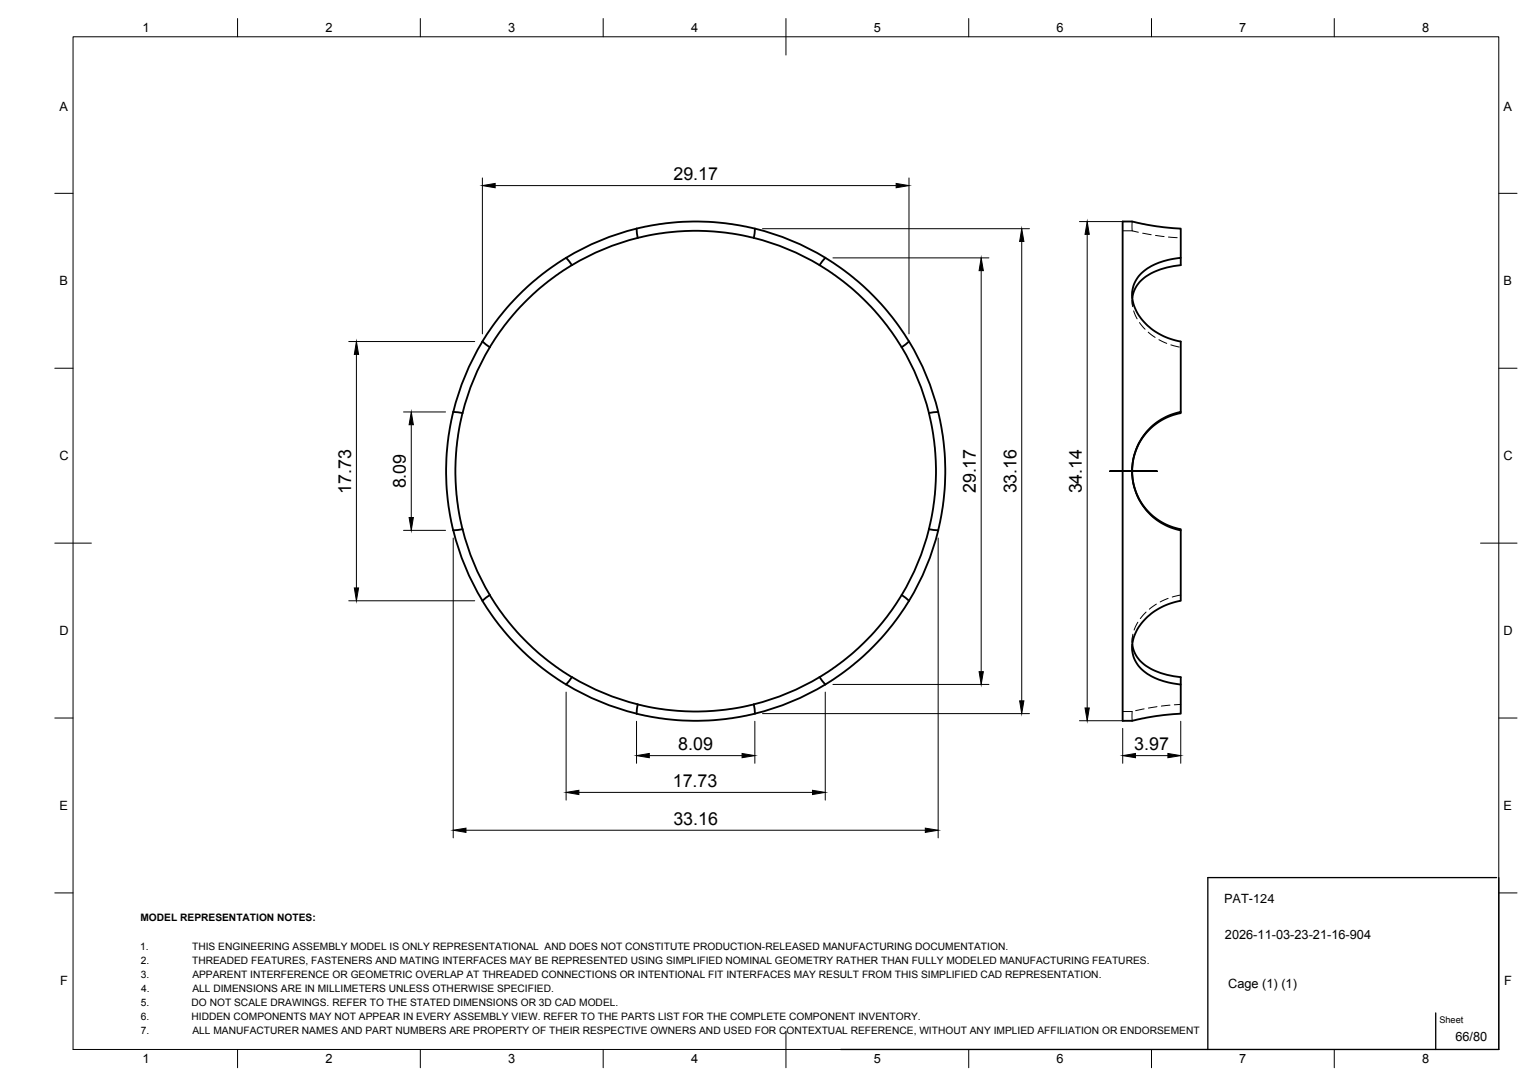
ISO-10303-21;
HEADER;
/* Generated by software containing ST-Developer
 * from STEP Tools, Inc. (www.steptools.com) 
 */

FILE_DESCRIPTION(
/* description */ ('XY cross-slide table'),
/* implementation_level */ '2;1');

FILE_NAME(
/* name */ 'Cage (1) (1).step',
/* time_stamp */ '2026-10-28T03:22:46-07:00',
/* author */ (''),
/* organization */ (''),
/* preprocessor_version */ 'ST-DEVELOPER v20.2',
/* originating_system */ 'Autodesk Translation Framework v15.17.0.0',
/* authorisation */ '');

FILE_SCHEMA (('AUTOMOTIVE_DESIGN { 1 0 10303 214 3 1 1 }'));
ENDSEC;

DATA;
#10=MECHANICAL_DESIGN_GEOMETRIC_PRESENTATION_REPRESENTATION('',(#1758),#62984);
#1051=B_SPLINE_CURVE_WITH_KNOTS('',3,(#49166,#49167,#49168,#49169,#49170,
#49171,#49172,#49173,#49174,#49175,#49176,#49177,#49178,#49179,#49180,#49181,
#49182,#49183,#49184,#49185,#49186,#49187),.UNSPECIFIED.,.F.,.F.,(4,2,2,
2,2,2,2,2,2,2,4),(0.0789094028588958,0.210573405340968,0.315860108011452,
0.421146810681936,0.522142632548711,0.623138454415485,0.72413427628226,
0.825130098149035,0.930416800819519,1.03570350349,1.16736750597208),
 .UNSPECIFIED.);
#1052=B_SPLINE_CURVE_WITH_KNOTS('',3,(#49191,#49192,#49193,#49194,#49195,
#49196,#49197,#49198,#49199,#49200,#49201,#49202,#49203,#49204,#49205,#49206,
#49207,#49208,#49209,#49210,#49211,#49212),.UNSPECIFIED.,.F.,.F.,(4,2,2,
2,2,2,2,2,2,2,4),(0.0774793363974613,0.142088896491891,0.284177792983782,
0.411119756996526,0.514392970548519,0.617666184100513,0.720939397652506,
0.8242126112045,0.951154575217244,1.09324347170913,1.15785303180356),
 .UNSPECIFIED.);
#1053=B_SPLINE_CURVE_WITH_KNOTS('',3,(#49218,#49219,#49220,#49221,#49222,
#49223,#49224,#49225,#49226,#49227,#49228,#49229,#49230,#49231,#49232,#49233,
#49234,#49235,#49236,#49237,#49238,#49239),.UNSPECIFIED.,.F.,.F.,(4,2,2,
2,2,2,2,2,2,2,4),(0.0774793363974613,0.142088896491891,0.284177792983782,
0.411119756996525,0.514392970548519,0.617666184100513,0.720939397652506,
0.8242126112045,0.951154575217243,1.09324347170913,1.15785303180356),
 .UNSPECIFIED.);
#1054=B_SPLINE_CURVE_WITH_KNOTS('',3,(#49243,#49244,#49245,#49246,#49247,
#49248,#49249,#49250,#49251,#49252,#49253,#49254,#49255,#49256,#49257,#49258,
#49259,#49260,#49261,#49262,#49263,#49264),.UNSPECIFIED.,.F.,.F.,(4,2,2,
2,2,2,2,2,2,2,4),(0.0774793363974614,0.142088896491891,0.284177792983781,
0.411119756996525,0.514392970548519,0.617666184100512,0.720939397652506,
0.824212611204499,0.951154575217243,1.09324347170913,1.15785303180356),
 .UNSPECIFIED.);
#1055=B_SPLINE_CURVE_WITH_KNOTS('',3,(#49268,#49269,#49270,#49271,#49272,
#49273,#49274,#49275,#49276,#49277,#49278,#49279),.UNSPECIFIED.,.F.,.F.,
(4,2,2,2,2,4),(0.0774793363974613,0.142088896491891,0.284177792983781,0.411119756996525,
0.514392970548519,0.617666184100512),.UNSPECIFIED.);
#1056=B_SPLINE_CURVE_WITH_KNOTS('',3,(#49284,#49285,#49286,#49287,#49288,
#49289,#49290,#49291,#49292,#49293,#49294,#49295),.UNSPECIFIED.,.F.,.F.,
(4,2,2,2,2,4),(0.617666184100512,0.720939397652506,0.824212611204499,0.951154575217243,
1.09324347170913,1.15785303180356),.UNSPECIFIED.);
#1057=B_SPLINE_CURVE_WITH_KNOTS('',3,(#49299,#49300,#49301,#49302,#49303,
#49304,#49305,#49306,#49307,#49308,#49309,#49310,#49311,#49312,#49313,#49314,
#49315,#49316,#49317,#49318,#49319,#49320),.UNSPECIFIED.,.F.,.F.,(4,2,2,
2,2,2,2,2,2,2,4),(0.0774793363974613,0.142088896491891,0.284177792983782,
0.411119756996526,0.514392970548519,0.617666184100513,0.720939397652507,
0.8242126112045,0.951154575217245,1.09324347170914,1.15785303180356),
 .UNSPECIFIED.);
#1058=B_SPLINE_CURVE_WITH_KNOTS('',3,(#49324,#49325,#49326,#49327,#49328,
#49329,#49330,#49331,#49332,#49333,#49334,#49335,#49336,#49337,#49338,#49339,
#49340,#49341,#49342,#49343,#49344,#49345),.UNSPECIFIED.,.F.,.F.,(4,2,2,
2,2,2,2,2,2,2,4),(0.0774793363974613,0.142088896491891,0.284177792983782,
0.411119756996526,0.514392970548519,0.617666184100513,0.720939397652506,
0.824212611204499,0.951154575217243,1.09324347170913,1.15785303180356),
 .UNSPECIFIED.);
#1059=B_SPLINE_CURVE_WITH_KNOTS('',3,(#49349,#49350,#49351,#49352,#49353,
#49354,#49355,#49356,#49357,#49358,#49359,#49360,#49361,#49362,#49363,#49364,
#49365,#49366,#49367,#49368,#49369,#49370),.UNSPECIFIED.,.F.,.F.,(4,2,2,
2,2,2,2,2,2,2,4),(0.0774793363974613,0.142088896491891,0.284177792983782,
0.411119756996526,0.514392970548519,0.617666184100513,0.720939397652506,
0.8242126112045,0.951154575217244,1.09324347170913,1.15785303180356),
 .UNSPECIFIED.);
#1060=B_SPLINE_CURVE_WITH_KNOTS('',3,(#49374,#49375,#49376,#49377,#49378,
#49379,#49380,#49381,#49382,#49383,#49384,#49385,#49386,#49387,#49388,#49389,
#49390,#49391,#49392,#49393,#49394,#49395),.UNSPECIFIED.,.F.,.F.,(4,2,2,
2,2,2,2,2,2,2,4),(0.0774793363974613,0.142088896491891,0.284177792983782,
0.411119756996526,0.514392970548519,0.617666184100513,0.720939397652506,
0.8242126112045,0.951154575217243,1.09324347170913,1.15785303180356),
 .UNSPECIFIED.);
#1061=B_SPLINE_CURVE_WITH_KNOTS('',3,(#49403,#49404,#49405,#49406,#49407,
#49408,#49409,#49410,#49411,#49412,#49413,#49414,#49415,#49416,#49417,#49418,
#49419,#49420,#49421,#49422,#49423,#49424),.UNSPECIFIED.,.F.,.F.,(4,2,2,
2,2,2,2,2,2,2,4),(0.0789094028588958,0.210573405340968,0.315860108011452,
0.421146810681936,0.522142632548711,0.623138454415485,0.72413427628226,
0.825130098149035,0.930416800819519,1.03570350349,1.16736750597208),
 .UNSPECIFIED.);
#1062=B_SPLINE_CURVE_WITH_KNOTS('',3,(#49432,#49433,#49434,#49435,#49436,
#49437,#49438,#49439,#49440,#49441,#49442,#49443,#49444,#49445,#49446,#49447,
#49448,#49449,#49450,#49451,#49452,#49453),.UNSPECIFIED.,.F.,.F.,(4,2,2,
2,2,2,2,2,2,2,4),(0.0789094028588958,0.210573405340969,0.315860108011453,
0.421146810681937,0.522142632548712,0.623138454415486,0.724134276282261,
0.825130098149035,0.930416800819519,1.03570350349,1.16736750597208),
 .UNSPECIFIED.);
#1063=B_SPLINE_CURVE_WITH_KNOTS('',3,(#49462,#49463,#49464,#49465,#49466,
#49467,#49468,#49469,#49470,#49471,#49472,#49473),.UNSPECIFIED.,.F.,.F.,
(4,2,2,2,2,4),(0.0789094028588958,0.210573405340968,0.315860108011452,0.421146810681937,
0.522142632548711,0.623138454415486),.UNSPECIFIED.);
#1064=B_SPLINE_CURVE_WITH_KNOTS('',3,(#49475,#49476,#49477,#49478,#49479,
#49480,#49481,#49482,#49483,#49484,#49485,#49486),.UNSPECIFIED.,.F.,.F.,
(4,2,2,2,2,4),(0.623138454415486,0.72413427628226,0.825130098149035,0.930416800819519,
1.03570350349,1.16736750597208),.UNSPECIFIED.);
#1065=B_SPLINE_CURVE_WITH_KNOTS('',3,(#49493,#49494,#49495,#49496,#49497,
#49498,#49499,#49500,#49501,#49502,#49503,#49504,#49505,#49506,#49507,#49508,
#49509,#49510,#49511,#49512,#49513,#49514),.UNSPECIFIED.,.F.,.F.,(4,2,2,
2,2,2,2,2,2,2,4),(0.0789094028588958,0.210573405340968,0.315860108011452,
0.421146810681936,0.522142632548711,0.623138454415486,0.72413427628226,
0.825130098149035,0.930416800819519,1.03570350349,1.16736750597208),
 .UNSPECIFIED.);
#1066=B_SPLINE_CURVE_WITH_KNOTS('',3,(#49522,#49523,#49524,#49525,#49526,
#49527,#49528,#49529,#49530,#49531,#49532,#49533,#49534,#49535,#49536,#49537,
#49538,#49539,#49540,#49541,#49542,#49543),.UNSPECIFIED.,.F.,.F.,(4,2,2,
2,2,2,2,2,2,2,4),(0.0789094028588957,0.210573405340968,0.315860108011452,
0.421146810681936,0.522142632548711,0.623138454415485,0.72413427628226,
0.825130098149035,0.930416800819519,1.03570350349,1.16736750597207),
 .UNSPECIFIED.);
#1067=B_SPLINE_CURVE_WITH_KNOTS('',3,(#49551,#49552,#49553,#49554,#49555,
#49556,#49557,#49558,#49559,#49560,#49561,#49562,#49563,#49564,#49565,#49566,
#49567,#49568,#49569,#49570,#49571,#49572),.UNSPECIFIED.,.F.,.F.,(4,2,2,
2,2,2,2,2,2,2,4),(0.0789094028588958,0.210573405340968,0.315860108011452,
0.421146810681936,0.522142632548711,0.623138454415486,0.72413427628226,
0.825130098149035,0.930416800819519,1.03570350349,1.16736750597208),
 .UNSPECIFIED.);
#1068=B_SPLINE_CURVE_WITH_KNOTS('',3,(#49581,#49582,#49583,#49584,#49585,
#49586,#49587,#49588,#49589,#49590,#49591,#49592,#49593,#49594,#49595,#49596,
#49597,#49598,#49599,#49600,#49601,#49602),.UNSPECIFIED.,.F.,.F.,(4,2,2,
2,2,2,2,2,2,2,4),(0.0789094028588958,0.210573405340968,0.315860108011452,
0.421146810681936,0.522142632548711,0.623138454415485,0.72413427628226,
0.825130098149035,0.930416800819519,1.03570350349,1.16736750597208),
 .UNSPECIFIED.);
#1433=SPHERICAL_SURFACE('',#25717,0.412776);
#1434=SPHERICAL_SURFACE('',#25733,0.412776);
#1435=SPHERICAL_SURFACE('',#25738,0.412776);
#1436=SPHERICAL_SURFACE('',#25743,0.412776);
#1437=SPHERICAL_SURFACE('',#25748,0.412776);
#1438=SPHERICAL_SURFACE('',#25753,0.412776);
#1439=SPHERICAL_SURFACE('',#25758,0.412776);
#1440=SPHERICAL_SURFACE('',#25766,0.412776);
#1563=SHAPE_REPRESENTATION_RELATIONSHIP('SRR','None',#63420,#1646);
#1646=ADVANCED_BREP_SHAPE_REPRESENTATION('',(#1867),#62957);
#1758=STYLED_ITEM('',(#63926),#1867);
#1867=MANIFOLD_SOLID_BREP('Continuous crown cage',#23056);
#2214=FACE_BOUND('',#5406,.T.);
#2682=PLANE('',#25730);
#2683=PLANE('',#25735);
#2684=PLANE('',#25740);
#2685=PLANE('',#25745);
#2686=PLANE('',#25750);
#2687=PLANE('',#25755);
#2688=PLANE('',#25764);
#2689=PLANE('',#25768);
#2690=PLANE('',#25769);
#3747=FACE_OUTER_BOUND('',#5388,.T.);
#3748=FACE_OUTER_BOUND('',#5389,.T.);
#3749=FACE_OUTER_BOUND('',#5390,.T.);
#3750=FACE_OUTER_BOUND('',#5391,.T.);
#3751=FACE_OUTER_BOUND('',#5392,.T.);
#3752=FACE_OUTER_BOUND('',#5393,.T.);
#3753=FACE_OUTER_BOUND('',#5394,.T.);
#3754=FACE_OUTER_BOUND('',#5395,.T.);
#3755=FACE_OUTER_BOUND('',#5396,.T.);
#3756=FACE_OUTER_BOUND('',#5397,.T.);
#3757=FACE_OUTER_BOUND('',#5398,.T.);
#3758=FACE_OUTER_BOUND('',#5399,.T.);
#3759=FACE_OUTER_BOUND('',#5400,.T.);
#3760=FACE_OUTER_BOUND('',#5401,.T.);
#3761=FACE_OUTER_BOUND('',#5402,.T.);
#3762=FACE_OUTER_BOUND('',#5403,.T.);
#3763=FACE_OUTER_BOUND('',#5404,.T.);
#3764=FACE_OUTER_BOUND('',#5405,.T.);
#3765=FACE_OUTER_BOUND('',#5407,.T.);
#5388=EDGE_LOOP('',(#18906,#18907,#18908,#18909));
#5389=EDGE_LOOP('',(#18910,#18911,#18912,#18913,#18914,#18915,#18916,#18917,
#18918,#18919,#18920,#18921,#18922,#18923,#18924,#18925,#18926,#18927,#18928,
#18929));
#5390=EDGE_LOOP('',(#18930,#18931,#18932,#18933));
#5391=EDGE_LOOP('',(#18934,#18935,#18936,#18937));
#5392=EDGE_LOOP('',(#18938,#18939,#18940,#18941));
#5393=EDGE_LOOP('',(#18942,#18943,#18944,#18945));
#5394=EDGE_LOOP('',(#18946,#18947,#18948,#18949));
#5395=EDGE_LOOP('',(#18950,#18951,#18952,#18953,#18954,#18955));
#5396=EDGE_LOOP('',(#18956,#18957,#18958,#18959));
#5397=EDGE_LOOP('',(#18960,#18961,#18962,#18963));
#5398=EDGE_LOOP('',(#18964,#18965,#18966,#18967));
#5399=EDGE_LOOP('',(#18968,#18969,#18970,#18971));
#5400=EDGE_LOOP('',(#18972,#18973,#18974,#18975));
#5401=EDGE_LOOP('',(#18976,#18977,#18978,#18979));
#5402=EDGE_LOOP('',(#18980,#18981,#18982,#18983,#18984,#18985,#18986,#18987,
#18988,#18989,#18990,#18991,#18992,#18993,#18994,#18995,#18996,#18997,#18998,
#18999));
#5403=EDGE_LOOP('',(#19000,#19001,#19002,#19003));
#5404=EDGE_LOOP('',(#19004,#19005,#19006,#19007));
#5405=EDGE_LOOP('',(#19008));
#5406=EDGE_LOOP('',(#19009));
#5407=EDGE_LOOP('',(#19010,#19011,#19012,#19013));
#6863=LINE('',#49281,#8350);
#6864=LINE('',#49577,#8351);
#8350=VECTOR('',#30866,1.706752);
#8351=VECTOR('',#30943,1.643248);
#9566=CIRCLE('',#25718,0.405071403305639);
#9567=CIRCLE('',#25719,0.405071403305639);
#9568=CIRCLE('',#25721,1.706752);
#9569=CIRCLE('',#25722,1.706752);
#9570=CIRCLE('',#25723,1.706752);
#9571=CIRCLE('',#25724,1.706752);
#9572=CIRCLE('',#25725,1.706752);
#9573=CIRCLE('',#25726,1.706752);
#9574=CIRCLE('',#25727,1.706752);
#9575=CIRCLE('',#25728,1.706752);
#9576=CIRCLE('',#25729,1.706752);
#9577=CIRCLE('',#25731,1.643248);
#9578=CIRCLE('',#25732,0.405071403305639);
#9579=CIRCLE('',#25734,0.405071403305639);
#9580=CIRCLE('',#25736,1.643248);
#9581=CIRCLE('',#25737,0.405071403305639);
#9582=CIRCLE('',#25739,0.405071403305639);
#9583=CIRCLE('',#25741,1.643248);
#9584=CIRCLE('',#25742,0.405071403305639);
#9585=CIRCLE('',#25744,0.405071403305639);
#9586=CIRCLE('',#25746,1.643248);
#9587=CIRCLE('',#25747,0.405071403305639);
#9588=CIRCLE('',#25749,0.405071403305639);
#9589=CIRCLE('',#25751,1.643248);
#9590=CIRCLE('',#25752,0.405071403305639);
#9591=CIRCLE('',#25754,0.405071403305639);
#9592=CIRCLE('',#25756,1.643248);
#9593=CIRCLE('',#25757,0.405071403305639);
#9594=CIRCLE('',#25759,0.405071403305639);
#9595=CIRCLE('',#25761,1.643248);
#9596=CIRCLE('',#25762,1.643248);
#9597=CIRCLE('',#25763,1.643248);
#9598=CIRCLE('',#25765,0.405071403305639);
#9599=CIRCLE('',#25767,0.405071403305639);
#11131=VERTEX_POINT('',#49164);
#11132=VERTEX_POINT('',#49165);
#11133=VERTEX_POINT('',#49188);
#11134=VERTEX_POINT('',#49190);
#11135=VERTEX_POINT('',#49215);
#11136=VERTEX_POINT('',#49217);
#11137=VERTEX_POINT('',#49240);
#11138=VERTEX_POINT('',#49242);
#11139=VERTEX_POINT('',#49265);
#11140=VERTEX_POINT('',#49267);
#11141=VERTEX_POINT('',#49280);
#11142=VERTEX_POINT('',#49283);
#11143=VERTEX_POINT('',#49296);
#11144=VERTEX_POINT('',#49298);
#11145=VERTEX_POINT('',#49321);
#11146=VERTEX_POINT('',#49323);
#11147=VERTEX_POINT('',#49346);
#11148=VERTEX_POINT('',#49348);
#11149=VERTEX_POINT('',#49371);
#11150=VERTEX_POINT('',#49373);
#11151=VERTEX_POINT('',#49398);
#11152=VERTEX_POINT('',#49402);
#11153=VERTEX_POINT('',#49427);
#11154=VERTEX_POINT('',#49431);
#11155=VERTEX_POINT('',#49456);
#11156=VERTEX_POINT('',#49460);
#11157=VERTEX_POINT('',#49461);
#11158=VERTEX_POINT('',#49488);
#11159=VERTEX_POINT('',#49492);
#11160=VERTEX_POINT('',#49517);
#11161=VERTEX_POINT('',#49521);
#11162=VERTEX_POINT('',#49546);
#11163=VERTEX_POINT('',#49550);
#11164=VERTEX_POINT('',#49575);
#11165=VERTEX_POINT('',#49578);
#11166=VERTEX_POINT('',#49580);
#13837=EDGE_CURVE('',#11131,#11132,#1051,.T.);
#13838=EDGE_CURVE('',#11133,#11131,#9566,.T.);
#13839=EDGE_CURVE('',#11134,#11133,#1052,.T.);
#13840=EDGE_CURVE('',#11132,#11134,#9567,.T.);
#13841=EDGE_CURVE('',#11135,#11133,#9568,.T.);
#13842=EDGE_CURVE('',#11135,#11136,#1053,.T.);
#13843=EDGE_CURVE('',#11137,#11136,#9569,.T.);
#13844=EDGE_CURVE('',#11137,#11138,#1054,.T.);
#13845=EDGE_CURVE('',#11139,#11138,#9570,.T.);
#13846=EDGE_CURVE('',#11139,#11140,#1055,.T.);
#13847=EDGE_CURVE('',#11140,#11141,#6863,.T.);
#13848=EDGE_CURVE('',#11141,#11141,#9571,.T.);
#13849=EDGE_CURVE('',#11140,#11142,#1056,.T.);
#13850=EDGE_CURVE('',#11143,#11142,#9572,.T.);
#13851=EDGE_CURVE('',#11143,#11144,#1057,.T.);
#13852=EDGE_CURVE('',#11145,#11144,#9573,.T.);
#13853=EDGE_CURVE('',#11145,#11146,#1058,.T.);
#13854=EDGE_CURVE('',#11147,#11146,#9574,.T.);
#13855=EDGE_CURVE('',#11147,#11148,#1059,.T.);
#13856=EDGE_CURVE('',#11149,#11148,#9575,.T.);
#13857=EDGE_CURVE('',#11149,#11150,#1060,.T.);
#13858=EDGE_CURVE('',#11134,#11150,#9576,.T.);
#13859=EDGE_CURVE('',#11131,#11151,#9577,.T.);
#13860=EDGE_CURVE('',#11151,#11135,#9578,.T.);
#13861=EDGE_CURVE('',#11152,#11151,#1061,.T.);
#13862=EDGE_CURVE('',#11136,#11152,#9579,.T.);
#13863=EDGE_CURVE('',#11152,#11153,#9580,.T.);
#13864=EDGE_CURVE('',#11153,#11137,#9581,.T.);
#13865=EDGE_CURVE('',#11154,#11153,#1062,.T.);
#13866=EDGE_CURVE('',#11138,#11154,#9582,.T.);
#13867=EDGE_CURVE('',#11154,#11155,#9583,.T.);
#13868=EDGE_CURVE('',#11155,#11139,#9584,.T.);
#13869=EDGE_CURVE('',#11156,#11157,#1063,.T.);
#13870=EDGE_CURVE('',#11142,#11156,#9585,.T.);
#13871=EDGE_CURVE('',#11157,#11155,#1064,.T.);
#13872=EDGE_CURVE('',#11156,#11158,#9586,.T.);
#13873=EDGE_CURVE('',#11158,#11143,#9587,.T.);
#13874=EDGE_CURVE('',#11159,#11158,#1065,.T.);
#13875=EDGE_CURVE('',#11144,#11159,#9588,.T.);
#13876=EDGE_CURVE('',#11159,#11160,#9589,.T.);
#13877=EDGE_CURVE('',#11160,#11145,#9590,.T.);
#13878=EDGE_CURVE('',#11161,#11160,#1066,.T.);
#13879=EDGE_CURVE('',#11146,#11161,#9591,.T.);
#13880=EDGE_CURVE('',#11161,#11162,#9592,.T.);
#13881=EDGE_CURVE('',#11162,#11147,#9593,.T.);
#13882=EDGE_CURVE('',#11163,#11162,#1067,.T.);
#13883=EDGE_CURVE('',#11148,#11163,#9594,.T.);
#13884=EDGE_CURVE('',#11164,#11164,#9595,.T.);
#13885=EDGE_CURVE('',#11164,#11157,#6864,.T.);
#13886=EDGE_CURVE('',#11165,#11132,#9596,.T.);
#13887=EDGE_CURVE('',#11165,#11166,#1068,.T.);
#13888=EDGE_CURVE('',#11163,#11166,#9597,.T.);
#13889=EDGE_CURVE('',#11150,#11165,#9598,.T.);
#13890=EDGE_CURVE('',#11166,#11149,#9599,.T.);
#18906=ORIENTED_EDGE('',*,*,#13837,.F.);
#18907=ORIENTED_EDGE('',*,*,#13838,.F.);
#18908=ORIENTED_EDGE('',*,*,#13839,.F.);
#18909=ORIENTED_EDGE('',*,*,#13840,.F.);
#18910=ORIENTED_EDGE('',*,*,#13839,.T.);
#18911=ORIENTED_EDGE('',*,*,#13841,.F.);
#18912=ORIENTED_EDGE('',*,*,#13842,.T.);
#18913=ORIENTED_EDGE('',*,*,#13843,.F.);
#18914=ORIENTED_EDGE('',*,*,#13844,.T.);
#18915=ORIENTED_EDGE('',*,*,#13845,.F.);
#18916=ORIENTED_EDGE('',*,*,#13846,.T.);
#18917=ORIENTED_EDGE('',*,*,#13847,.T.);
#18918=ORIENTED_EDGE('',*,*,#13848,.F.);
#18919=ORIENTED_EDGE('',*,*,#13847,.F.);
#18920=ORIENTED_EDGE('',*,*,#13849,.T.);
#18921=ORIENTED_EDGE('',*,*,#13850,.F.);
#18922=ORIENTED_EDGE('',*,*,#13851,.T.);
#18923=ORIENTED_EDGE('',*,*,#13852,.F.);
#18924=ORIENTED_EDGE('',*,*,#13853,.T.);
#18925=ORIENTED_EDGE('',*,*,#13854,.F.);
#18926=ORIENTED_EDGE('',*,*,#13855,.T.);
#18927=ORIENTED_EDGE('',*,*,#13856,.F.);
#18928=ORIENTED_EDGE('',*,*,#13857,.T.);
#18929=ORIENTED_EDGE('',*,*,#13858,.F.);
#18930=ORIENTED_EDGE('',*,*,#13838,.T.);
#18931=ORIENTED_EDGE('',*,*,#13859,.T.);
#18932=ORIENTED_EDGE('',*,*,#13860,.T.);
#18933=ORIENTED_EDGE('',*,*,#13841,.T.);
#18934=ORIENTED_EDGE('',*,*,#13861,.F.);
#18935=ORIENTED_EDGE('',*,*,#13862,.F.);
#18936=ORIENTED_EDGE('',*,*,#13842,.F.);
#18937=ORIENTED_EDGE('',*,*,#13860,.F.);
#18938=ORIENTED_EDGE('',*,*,#13862,.T.);
#18939=ORIENTED_EDGE('',*,*,#13863,.T.);
#18940=ORIENTED_EDGE('',*,*,#13864,.T.);
#18941=ORIENTED_EDGE('',*,*,#13843,.T.);
#18942=ORIENTED_EDGE('',*,*,#13865,.F.);
#18943=ORIENTED_EDGE('',*,*,#13866,.F.);
#18944=ORIENTED_EDGE('',*,*,#13844,.F.);
#18945=ORIENTED_EDGE('',*,*,#13864,.F.);
#18946=ORIENTED_EDGE('',*,*,#13866,.T.);
#18947=ORIENTED_EDGE('',*,*,#13867,.T.);
#18948=ORIENTED_EDGE('',*,*,#13868,.T.);
#18949=ORIENTED_EDGE('',*,*,#13845,.T.);
#18950=ORIENTED_EDGE('',*,*,#13869,.F.);
#18951=ORIENTED_EDGE('',*,*,#13870,.F.);
#18952=ORIENTED_EDGE('',*,*,#13849,.F.);
#18953=ORIENTED_EDGE('',*,*,#13846,.F.);
#18954=ORIENTED_EDGE('',*,*,#13868,.F.);
#18955=ORIENTED_EDGE('',*,*,#13871,.F.);
#18956=ORIENTED_EDGE('',*,*,#13870,.T.);
#18957=ORIENTED_EDGE('',*,*,#13872,.T.);
#18958=ORIENTED_EDGE('',*,*,#13873,.T.);
#18959=ORIENTED_EDGE('',*,*,#13850,.T.);
#18960=ORIENTED_EDGE('',*,*,#13874,.F.);
#18961=ORIENTED_EDGE('',*,*,#13875,.F.);
#18962=ORIENTED_EDGE('',*,*,#13851,.F.);
#18963=ORIENTED_EDGE('',*,*,#13873,.F.);
#18964=ORIENTED_EDGE('',*,*,#13875,.T.);
#18965=ORIENTED_EDGE('',*,*,#13876,.T.);
#18966=ORIENTED_EDGE('',*,*,#13877,.T.);
#18967=ORIENTED_EDGE('',*,*,#13852,.T.);
#18968=ORIENTED_EDGE('',*,*,#13878,.F.);
#18969=ORIENTED_EDGE('',*,*,#13879,.F.);
#18970=ORIENTED_EDGE('',*,*,#13853,.F.);
#18971=ORIENTED_EDGE('',*,*,#13877,.F.);
#18972=ORIENTED_EDGE('',*,*,#13879,.T.);
#18973=ORIENTED_EDGE('',*,*,#13880,.T.);
#18974=ORIENTED_EDGE('',*,*,#13881,.T.);
#18975=ORIENTED_EDGE('',*,*,#13854,.T.);
#18976=ORIENTED_EDGE('',*,*,#13855,.F.);
#18977=ORIENTED_EDGE('',*,*,#13881,.F.);
#18978=ORIENTED_EDGE('',*,*,#13882,.F.);
#18979=ORIENTED_EDGE('',*,*,#13883,.F.);
#18980=ORIENTED_EDGE('',*,*,#13884,.F.);
#18981=ORIENTED_EDGE('',*,*,#13885,.T.);
#18982=ORIENTED_EDGE('',*,*,#13871,.T.);
#18983=ORIENTED_EDGE('',*,*,#13867,.F.);
#18984=ORIENTED_EDGE('',*,*,#13865,.T.);
#18985=ORIENTED_EDGE('',*,*,#13863,.F.);
#18986=ORIENTED_EDGE('',*,*,#13861,.T.);
#18987=ORIENTED_EDGE('',*,*,#13859,.F.);
#18988=ORIENTED_EDGE('',*,*,#13837,.T.);
#18989=ORIENTED_EDGE('',*,*,#13886,.F.);
#18990=ORIENTED_EDGE('',*,*,#13887,.T.);
#18991=ORIENTED_EDGE('',*,*,#13888,.F.);
#18992=ORIENTED_EDGE('',*,*,#13882,.T.);
#18993=ORIENTED_EDGE('',*,*,#13880,.F.);
#18994=ORIENTED_EDGE('',*,*,#13878,.T.);
#18995=ORIENTED_EDGE('',*,*,#13876,.F.);
#18996=ORIENTED_EDGE('',*,*,#13874,.T.);
#18997=ORIENTED_EDGE('',*,*,#13872,.F.);
#18998=ORIENTED_EDGE('',*,*,#13869,.T.);
#18999=ORIENTED_EDGE('',*,*,#13885,.F.);
#19000=ORIENTED_EDGE('',*,*,#13840,.T.);
#19001=ORIENTED_EDGE('',*,*,#13858,.T.);
#19002=ORIENTED_EDGE('',*,*,#13889,.T.);
#19003=ORIENTED_EDGE('',*,*,#13886,.T.);
#19004=ORIENTED_EDGE('',*,*,#13857,.F.);
#19005=ORIENTED_EDGE('',*,*,#13890,.F.);
#19006=ORIENTED_EDGE('',*,*,#13887,.F.);
#19007=ORIENTED_EDGE('',*,*,#13889,.F.);
#19008=ORIENTED_EDGE('',*,*,#13848,.T.);
#19009=ORIENTED_EDGE('',*,*,#13884,.T.);
#19010=ORIENTED_EDGE('',*,*,#13883,.T.);
#19011=ORIENTED_EDGE('',*,*,#13888,.T.);
#19012=ORIENTED_EDGE('',*,*,#13890,.T.);
#19013=ORIENTED_EDGE('',*,*,#13856,.T.);
#21434=CYLINDRICAL_SURFACE('',#25720,1.706752);
#21435=CYLINDRICAL_SURFACE('',#25760,1.643248);
#22528=ADVANCED_FACE('',(#3747),#1433,.F.);
#22529=ADVANCED_FACE('',(#3748),#21434,.T.);
#22530=ADVANCED_FACE('',(#3749),#2682,.T.);
#22531=ADVANCED_FACE('',(#3750),#1434,.F.);
#22532=ADVANCED_FACE('',(#3751),#2683,.T.);
#22533=ADVANCED_FACE('',(#3752),#1435,.F.);
#22534=ADVANCED_FACE('',(#3753),#2684,.T.);
#22535=ADVANCED_FACE('',(#3754),#1436,.F.);
#22536=ADVANCED_FACE('',(#3755),#2685,.T.);
#22537=ADVANCED_FACE('',(#3756),#1437,.F.);
#22538=ADVANCED_FACE('',(#3757),#2686,.T.);
#22539=ADVANCED_FACE('',(#3758),#1438,.F.);
#22540=ADVANCED_FACE('',(#3759),#2687,.T.);
#22541=ADVANCED_FACE('',(#3760),#1439,.F.);
#22542=ADVANCED_FACE('',(#3761),#21435,.F.);
#22543=ADVANCED_FACE('',(#3762),#2688,.T.);
#22544=ADVANCED_FACE('',(#3763),#1440,.F.);
#22545=ADVANCED_FACE('',(#3764,#2214),#2689,.T.);
#22546=ADVANCED_FACE('',(#3765),#2690,.T.);
#23056=CLOSED_SHELL('',(#22528,#22529,#22530,#22531,#22532,#22533,#22534,
#22535,#22536,#22537,#22538,#22539,#22540,#22541,#22542,#22543,#22544,#22545,
#22546));
#25716=AXIS2_PLACEMENT_3D('',#49162,#30850,#30851);
#25717=AXIS2_PLACEMENT_3D('',#49163,#30852,#30853);
#25718=AXIS2_PLACEMENT_3D('',#49189,#30854,#30855);
#25719=AXIS2_PLACEMENT_3D('',#49213,#30856,#30857);
#25720=AXIS2_PLACEMENT_3D('',#49214,#30858,#30859);
#25721=AXIS2_PLACEMENT_3D('',#49216,#30860,#30861);
#25722=AXIS2_PLACEMENT_3D('',#49241,#30862,#30863);
#25723=AXIS2_PLACEMENT_3D('',#49266,#30864,#30865);
#25724=AXIS2_PLACEMENT_3D('',#49282,#30867,#30868);
#25725=AXIS2_PLACEMENT_3D('',#49297,#30869,#30870);
#25726=AXIS2_PLACEMENT_3D('',#49322,#30871,#30872);
#25727=AXIS2_PLACEMENT_3D('',#49347,#30873,#30874);
#25728=AXIS2_PLACEMENT_3D('',#49372,#30875,#30876);
#25729=AXIS2_PLACEMENT_3D('',#49396,#30877,#30878);
#25730=AXIS2_PLACEMENT_3D('',#49397,#30879,#30880);
#25731=AXIS2_PLACEMENT_3D('',#49399,#30881,#30882);
#25732=AXIS2_PLACEMENT_3D('',#49400,#30883,#30884);
#25733=AXIS2_PLACEMENT_3D('',#49401,#30885,#30886);
#25734=AXIS2_PLACEMENT_3D('',#49425,#30887,#30888);
#25735=AXIS2_PLACEMENT_3D('',#49426,#30889,#30890);
#25736=AXIS2_PLACEMENT_3D('',#49428,#30891,#30892);
#25737=AXIS2_PLACEMENT_3D('',#49429,#30893,#30894);
#25738=AXIS2_PLACEMENT_3D('',#49430,#30895,#30896);
#25739=AXIS2_PLACEMENT_3D('',#49454,#30897,#30898);
#25740=AXIS2_PLACEMENT_3D('',#49455,#30899,#30900);
#25741=AXIS2_PLACEMENT_3D('',#49457,#30901,#30902);
#25742=AXIS2_PLACEMENT_3D('',#49458,#30903,#30904);
#25743=AXIS2_PLACEMENT_3D('',#49459,#30905,#30906);
#25744=AXIS2_PLACEMENT_3D('',#49474,#30907,#30908);
#25745=AXIS2_PLACEMENT_3D('',#49487,#30909,#30910);
#25746=AXIS2_PLACEMENT_3D('',#49489,#30911,#30912);
#25747=AXIS2_PLACEMENT_3D('',#49490,#30913,#30914);
#25748=AXIS2_PLACEMENT_3D('',#49491,#30915,#30916);
#25749=AXIS2_PLACEMENT_3D('',#49515,#30917,#30918);
#25750=AXIS2_PLACEMENT_3D('',#49516,#30919,#30920);
#25751=AXIS2_PLACEMENT_3D('',#49518,#30921,#30922);
#25752=AXIS2_PLACEMENT_3D('',#49519,#30923,#30924);
#25753=AXIS2_PLACEMENT_3D('',#49520,#30925,#30926);
#25754=AXIS2_PLACEMENT_3D('',#49544,#30927,#30928);
#25755=AXIS2_PLACEMENT_3D('',#49545,#30929,#30930);
#25756=AXIS2_PLACEMENT_3D('',#49547,#30931,#30932);
#25757=AXIS2_PLACEMENT_3D('',#49548,#30933,#30934);
#25758=AXIS2_PLACEMENT_3D('',#49549,#30935,#30936);
#25759=AXIS2_PLACEMENT_3D('',#49573,#30937,#30938);
#25760=AXIS2_PLACEMENT_3D('',#49574,#30939,#30940);
#25761=AXIS2_PLACEMENT_3D('',#49576,#30941,#30942);
#25762=AXIS2_PLACEMENT_3D('',#49579,#30944,#30945);
#25763=AXIS2_PLACEMENT_3D('',#49603,#30946,#30947);
#25764=AXIS2_PLACEMENT_3D('',#49604,#30948,#30949);
#25765=AXIS2_PLACEMENT_3D('',#49605,#30950,#30951);
#25766=AXIS2_PLACEMENT_3D('',#49606,#30952,#30953);
#25767=AXIS2_PLACEMENT_3D('',#49607,#30954,#30955);
#25768=AXIS2_PLACEMENT_3D('',#49608,#30956,#30957);
#25769=AXIS2_PLACEMENT_3D('',#49609,#30958,#30959);
#30850=DIRECTION('axis',(0.,0.,1.));
#30851=DIRECTION('refdir',(1.,0.,0.));
#30852=DIRECTION('center_axis',(0.,0.,1.));
#30853=DIRECTION('ref_axis',(1.,0.,0.));
#30854=DIRECTION('center_axis',(0.,-1.,0.));
#30855=DIRECTION('ref_axis',(0.,0.,-1.));
#30856=DIRECTION('center_axis',(0.,-1.,0.));
#30857=DIRECTION('ref_axis',(0.,0.,-1.));
#30858=DIRECTION('center_axis',(0.,1.,0.));
#30859=DIRECTION('ref_axis',(1.,0.,0.));
#30860=DIRECTION('center_axis',(0.,1.,0.));
#30861=DIRECTION('ref_axis',(1.,0.,0.));
#30862=DIRECTION('center_axis',(0.,1.,0.));
#30863=DIRECTION('ref_axis',(1.,0.,0.));
#30864=DIRECTION('center_axis',(0.,1.,0.));
#30865=DIRECTION('ref_axis',(1.,0.,0.));
#30866=DIRECTION('',(0.,-1.,0.));
#30867=DIRECTION('center_axis',(0.,-1.,0.));
#30868=DIRECTION('ref_axis',(1.,0.,0.));
#30869=DIRECTION('center_axis',(0.,1.,0.));
#30870=DIRECTION('ref_axis',(1.,0.,0.));
#30871=DIRECTION('center_axis',(0.,1.,0.));
#30872=DIRECTION('ref_axis',(1.,0.,0.));
#30873=DIRECTION('center_axis',(0.,1.,0.));
#30874=DIRECTION('ref_axis',(1.,0.,0.));
#30875=DIRECTION('center_axis',(0.,1.,0.));
#30876=DIRECTION('ref_axis',(1.,0.,0.));
#30877=DIRECTION('center_axis',(0.,1.,0.));
#30878=DIRECTION('ref_axis',(1.,0.,0.));
#30879=DIRECTION('center_axis',(0.,1.,0.));
#30880=DIRECTION('ref_axis',(1.,0.,0.));
#30881=DIRECTION('center_axis',(0.,-1.,0.));
#30882=DIRECTION('ref_axis',(1.,0.,0.));
#30883=DIRECTION('center_axis',(0.,-1.,0.));
#30884=DIRECTION('ref_axis',(0.,0.,-1.));
#30885=DIRECTION('center_axis',(6.12323399573677E-17,0.,1.));
#30886=DIRECTION('ref_axis',(1.,0.,0.));
#30887=DIRECTION('center_axis',(0.,-1.,0.));
#30888=DIRECTION('ref_axis',(0.,0.,-1.));
#30889=DIRECTION('center_axis',(0.,1.,0.));
#30890=DIRECTION('ref_axis',(1.,0.,0.));
#30891=DIRECTION('center_axis',(0.,-1.,0.));
#30892=DIRECTION('ref_axis',(1.,0.,0.));
#30893=DIRECTION('center_axis',(0.,-1.,0.));
#30894=DIRECTION('ref_axis',(0.,0.,-1.));
#30895=DIRECTION('center_axis',(0.,0.,1.));
#30896=DIRECTION('ref_axis',(1.,0.,0.));
#30897=DIRECTION('center_axis',(0.,-1.,0.));
#30898=DIRECTION('ref_axis',(0.,0.,-1.));
#30899=DIRECTION('center_axis',(0.,1.,0.));
#30900=DIRECTION('ref_axis',(1.,0.,0.));
#30901=DIRECTION('center_axis',(0.,-1.,0.));
#30902=DIRECTION('ref_axis',(1.,0.,0.));
#30903=DIRECTION('center_axis',(0.,-1.,0.));
#30904=DIRECTION('ref_axis',(0.,0.,-1.));
#30905=DIRECTION('center_axis',(0.,0.,1.));
#30906=DIRECTION('ref_axis',(1.,0.,0.));
#30907=DIRECTION('center_axis',(0.,-1.,0.));
#30908=DIRECTION('ref_axis',(0.,0.,-1.));
#30909=DIRECTION('center_axis',(0.,1.,0.));
#30910=DIRECTION('ref_axis',(1.,0.,0.));
#30911=DIRECTION('center_axis',(0.,-1.,0.));
#30912=DIRECTION('ref_axis',(1.,0.,0.));
#30913=DIRECTION('center_axis',(0.,-1.,0.));
#30914=DIRECTION('ref_axis',(0.,0.,-1.));
#30915=DIRECTION('center_axis',(0.,0.,1.));
#30916=DIRECTION('ref_axis',(1.,0.,0.));
#30917=DIRECTION('center_axis',(0.,-1.,0.));
#30918=DIRECTION('ref_axis',(0.,0.,-1.));
#30919=DIRECTION('center_axis',(0.,1.,0.));
#30920=DIRECTION('ref_axis',(1.,0.,0.));
#30921=DIRECTION('center_axis',(0.,-1.,0.));
#30922=DIRECTION('ref_axis',(1.,0.,0.));
#30923=DIRECTION('center_axis',(0.,-1.,0.));
#30924=DIRECTION('ref_axis',(0.,0.,-1.));
#30925=DIRECTION('center_axis',(6.12323399573676E-17,0.,1.));
#30926=DIRECTION('ref_axis',(1.,0.,0.));
#30927=DIRECTION('center_axis',(0.,-1.,0.));
#30928=DIRECTION('ref_axis',(0.,0.,-1.));
#30929=DIRECTION('center_axis',(0.,1.,0.));
#30930=DIRECTION('ref_axis',(1.,0.,0.));
#30931=DIRECTION('center_axis',(0.,-1.,0.));
#30932=DIRECTION('ref_axis',(1.,0.,0.));
#30933=DIRECTION('center_axis',(0.,-1.,0.));
#30934=DIRECTION('ref_axis',(0.,0.,-1.));
#30935=DIRECTION('center_axis',(0.,0.,1.));
#30936=DIRECTION('ref_axis',(1.,0.,0.));
#30937=DIRECTION('center_axis',(0.,-1.,0.));
#30938=DIRECTION('ref_axis',(0.,0.,-1.));
#30939=DIRECTION('center_axis',(0.,1.,0.));
#30940=DIRECTION('ref_axis',(1.,0.,0.));
#30941=DIRECTION('center_axis',(0.,1.,0.));
#30942=DIRECTION('ref_axis',(1.,0.,0.));
#30943=DIRECTION('',(0.,1.,0.));
#30944=DIRECTION('center_axis',(0.,-1.,0.));
#30945=DIRECTION('ref_axis',(1.,0.,0.));
#30946=DIRECTION('center_axis',(0.,-1.,0.));
#30947=DIRECTION('ref_axis',(1.,0.,0.));
#30948=DIRECTION('center_axis',(0.,1.,0.));
#30949=DIRECTION('ref_axis',(1.,0.,0.));
#30950=DIRECTION('center_axis',(0.,-1.,0.));
#30951=DIRECTION('ref_axis',(0.,0.,-1.));
#30952=DIRECTION('center_axis',(0.,0.,1.));
#30953=DIRECTION('ref_axis',(1.,0.,0.));
#30954=DIRECTION('center_axis',(0.,-1.,0.));
#30955=DIRECTION('ref_axis',(0.,0.,-1.));
#30956=DIRECTION('center_axis',(0.,-1.,0.));
#30957=DIRECTION('ref_axis',(-1.,0.,0.));
#30958=DIRECTION('center_axis',(0.,1.,0.));
#30959=DIRECTION('ref_axis',(1.,0.,0.));
#49162=CARTESIAN_POINT('',(0.,0.,0.));
#49163=CARTESIAN_POINT('Origin',(1.18440385848747,0.,1.18440385848747));
#49164=CARTESIAN_POINT('',(0.846804978391753,-0.07938,1.40825612658882));
#49165=CARTESIAN_POINT('',(1.40825612658882,-0.07938,0.846804978391754));
#49166=CARTESIAN_POINT('Ctrl Pts',(0.846804978391752,-0.0793800000000001,
1.40825612658882));
#49167=CARTESIAN_POINT('Ctrl Pts',(0.854205272175554,-0.123401821157026,
1.40380622184538));
#49168=CARTESIAN_POINT('Ctrl Pts',(0.867957148219441,-0.166543350814306,
1.39550172959303));
#49169=CARTESIAN_POINT('Ctrl Pts',(0.902193646979982,-0.237231147975234,
1.3735491215176));
#49170=CARTESIAN_POINT('Ctrl Pts',(0.920778333482564,-0.266264900654909,
1.36127834356734));
#49171=CARTESIAN_POINT('Ctrl Pts',(0.962485392528369,-0.317195968905306,
1.33211611256184));
#49172=CARTESIAN_POINT('Ctrl Pts',(0.985600426557816,-0.33909093068465,
1.31521005565926));
#49173=CARTESIAN_POINT('Ctrl Pts',(1.03253285680459,-0.373586846396559,
1.27866649102984));
#49174=CARTESIAN_POINT('Ctrl Pts',(1.05871835910697,-0.388086240756494,
1.25722555095714));
#49175=CARTESIAN_POINT('Ctrl Pts',(1.11153475808518,-0.407068917407805,
1.2107812086231));
#49176=CARTESIAN_POINT('Ctrl Pts',(1.13814686046673,-0.411552957311693,
1.18575674747573));
#49177=CARTESIAN_POINT('Ctrl Pts',(1.18575674747573,-0.411552957311693,
1.13814686046673));
#49178=CARTESIAN_POINT('Ctrl Pts',(1.2107812086231,-0.407068917407805,1.11153475808518));
#49179=CARTESIAN_POINT('Ctrl Pts',(1.25722555095713,-0.388086240756494,
1.05871835910697));
#49180=CARTESIAN_POINT('Ctrl Pts',(1.27866649102984,-0.373586846396559,
1.03253285680459));
#49181=CARTESIAN_POINT('Ctrl Pts',(1.31521005565926,-0.33909093068465,0.985600426557816));
#49182=CARTESIAN_POINT('Ctrl Pts',(1.33211611256184,-0.317195968905306,
0.962485392528369));
#49183=CARTESIAN_POINT('Ctrl Pts',(1.36127834356734,-0.266264900654909,
0.920778333482565));
#49184=CARTESIAN_POINT('Ctrl Pts',(1.3735491215176,-0.237231147975234,0.902193646979983));
#49185=CARTESIAN_POINT('Ctrl Pts',(1.39550172959303,-0.166543350814306,
0.867957148219442));
#49186=CARTESIAN_POINT('Ctrl Pts',(1.40380622184538,-0.123401821157026,
0.854205272175555));
#49187=CARTESIAN_POINT('Ctrl Pts',(1.40825612658882,-0.0793800000000001,
0.846804978391753));
#49188=CARTESIAN_POINT('',(0.886256117232623,-0.07938,1.45861320581289));
#49189=CARTESIAN_POINT('Origin',(1.18440385848747,-0.07938,1.18440385848747));
#49190=CARTESIAN_POINT('',(1.45861320581289,-0.07938,0.886256117232624));
#49191=CARTESIAN_POINT('Ctrl Pts',(1.45861320581289,-0.0793800000000001,
0.886256117232623));
#49192=CARTESIAN_POINT('Ctrl Pts',(1.45630208793976,-0.101649918886749,
0.890059788636852));
#49193=CARTESIAN_POINT('Ctrl Pts',(1.45296717977858,-0.123823518623746,
0.895520212222107));
#49194=CARTESIAN_POINT('Ctrl Pts',(1.43904931717599,-0.192480977588836,
0.917859913453975));
#49195=CARTESIAN_POINT('Ctrl Pts',(1.4243271592157,-0.236152929235938,0.940896403863072));
#49196=CARTESIAN_POINT('Ctrl Pts',(1.39055359345152,-0.303141259068212,
0.990027513266106));
#49197=CARTESIAN_POINT('Ctrl Pts',(1.36743459453896,-0.335108247315849,
1.02199477007745));
#49198=CARTESIAN_POINT('Ctrl Pts',(1.32643091652006,-0.373243761060364,
1.07446535104584));
#49199=CARTESIAN_POINT('Ctrl Pts',(1.30441816675528,-0.387888272594439,
1.10126842659597));
#49200=CARTESIAN_POINT('Ctrl Pts',(1.25681160160691,-0.407041111792943,
1.15530234155453));
#49201=CARTESIAN_POINT('Ctrl Pts',(1.23119764287622,-0.411552957311693,
1.18251418313119));
#49202=CARTESIAN_POINT('Ctrl Pts',(1.18251418313119,-0.411552957311693,
1.23119764287622));
#49203=CARTESIAN_POINT('Ctrl Pts',(1.15530234155453,-0.407041111792943,
1.25681160160691));
#49204=CARTESIAN_POINT('Ctrl Pts',(1.10126842659597,-0.387888272594439,
1.30441816675528));
#49205=CARTESIAN_POINT('Ctrl Pts',(1.07446535104584,-0.373243761060364,
1.32643091652006));
#49206=CARTESIAN_POINT('Ctrl Pts',(1.02199477007745,-0.335108247315848,
1.36743459453896));
#49207=CARTESIAN_POINT('Ctrl Pts',(0.990027513266105,-0.303141259068211,
1.39055359345152));
#49208=CARTESIAN_POINT('Ctrl Pts',(0.940896403863071,-0.236152929235937,
1.42432715921571));
#49209=CARTESIAN_POINT('Ctrl Pts',(0.917859913453974,-0.192480977588835,
1.43904931717599));
#49210=CARTESIAN_POINT('Ctrl Pts',(0.895520212222106,-0.123823518623745,
1.45296717977858));
#49211=CARTESIAN_POINT('Ctrl Pts',(0.890059788636851,-0.101649918886749,
1.45630208793976));
#49212=CARTESIAN_POINT('Ctrl Pts',(0.886256117232622,-0.0793800000000001,
1.45861320581289));
#49213=CARTESIAN_POINT('Origin',(1.18440385848747,-0.07938,1.18440385848747));
#49214=CARTESIAN_POINT('Origin',(0.,-0.27783,0.));
#49215=CARTESIAN_POINT('',(0.404717578595295,-0.07938,1.65807299932179));
#49216=CARTESIAN_POINT('Origin',(0.,-0.07938,0.));
#49217=CARTESIAN_POINT('',(-0.404717578595296,-0.07938,1.65807299932179));
#49218=CARTESIAN_POINT('Ctrl Pts',(0.404717578595296,-0.0793800000000001,
1.65807299932179));
#49219=CARTESIAN_POINT('Ctrl Pts',(0.400393769631747,-0.101649918886749,
1.65912839404491));
#49220=CARTESIAN_POINT('Ctrl Pts',(0.394174530911058,-0.123823518623745,
1.66063136041479));
#49221=CARTESIAN_POINT('Ctrl Pts',(0.368536561654407,-0.192480977588835,
1.66658649961961));
#49222=CARTESIAN_POINT('Ctrl Pts',(0.341837165343982,-0.236152929235937,
1.67246562047521));
#49223=CARTESIAN_POINT('Ctrl Pts',(0.283214707341173,-0.303141259068211,
1.68332504372461));
#49224=CARTESIAN_POINT('Ctrl Pts',(0.244262842368623,-0.335108247315849,
1.68958170688653));
#49225=CARTESIAN_POINT('Ctrl Pts',(0.178166559972324,-0.373243761060364,
1.69769003172132));
#49226=CARTESIAN_POINT('Ctrl Pts',(0.143648558862931,-0.387888272594439,
1.70107730356824));
#49227=CARTESIAN_POINT('Ctrl Pts',(0.0717778861362652,-0.407041111792943,
1.70562212620408));
#49228=CARTESIAN_POINT('Ctrl Pts',(0.0344244045173309,-0.411552957311693,
1.706752));
#49229=CARTESIAN_POINT('Ctrl Pts',(-0.0344244045173315,-0.411552957311693,
1.706752));
#49230=CARTESIAN_POINT('Ctrl Pts',(-0.0717778861362658,-0.407041111792943,
1.70562212620408));
#49231=CARTESIAN_POINT('Ctrl Pts',(-0.143648558862932,-0.387888272594439,
1.70107730356824));
#49232=CARTESIAN_POINT('Ctrl Pts',(-0.178166559972325,-0.373243761060364,
1.69769003172132));
#49233=CARTESIAN_POINT('Ctrl Pts',(-0.244262842368624,-0.335108247315849,
1.68958170688653));
#49234=CARTESIAN_POINT('Ctrl Pts',(-0.283214707341173,-0.303141259068212,
1.68332504372461));
#49235=CARTESIAN_POINT('Ctrl Pts',(-0.341837165343982,-0.236152929235937,
1.67246562047521));
#49236=CARTESIAN_POINT('Ctrl Pts',(-0.368536561654408,-0.192480977588835,
1.66658649961961));
#49237=CARTESIAN_POINT('Ctrl Pts',(-0.394174530911059,-0.123823518623745,
1.66063136041479));
#49238=CARTESIAN_POINT('Ctrl Pts',(-0.400393769631748,-0.101649918886749,
1.65912839404491));
#49239=CARTESIAN_POINT('Ctrl Pts',(-0.404717578595297,-0.0793800000000001,
1.65807299932179));
#49240=CARTESIAN_POINT('',(-0.886256117232624,-0.07938,1.45861320581289));
#49241=CARTESIAN_POINT('Origin',(0.,-0.07938,0.));
#49242=CARTESIAN_POINT('',(-1.45861320581289,-0.07938,0.886256117232623));
#49243=CARTESIAN_POINT('Ctrl Pts',(-0.886256117232623,-0.0793800000000001,
1.45861320581289));
#49244=CARTESIAN_POINT('Ctrl Pts',(-0.890059788636852,-0.101649918886749,
1.45630208793976));
#49245=CARTESIAN_POINT('Ctrl Pts',(-0.895520212222106,-0.123823518623745,
1.45296717977858));
#49246=CARTESIAN_POINT('Ctrl Pts',(-0.917859913453974,-0.192480977588835,
1.43904931717599));
#49247=CARTESIAN_POINT('Ctrl Pts',(-0.940896403863071,-0.236152929235937,
1.4243271592157));
#49248=CARTESIAN_POINT('Ctrl Pts',(-0.990027513266105,-0.303141259068211,
1.39055359345152));
#49249=CARTESIAN_POINT('Ctrl Pts',(-1.02199477007745,-0.335108247315848,
1.36743459453896));
#49250=CARTESIAN_POINT('Ctrl Pts',(-1.07446535104584,-0.373243761060364,
1.32643091652006));
#49251=CARTESIAN_POINT('Ctrl Pts',(-1.10126842659597,-0.387888272594439,
1.30441816675528));
#49252=CARTESIAN_POINT('Ctrl Pts',(-1.15530234155453,-0.407041111792943,
1.25681160160691));
#49253=CARTESIAN_POINT('Ctrl Pts',(-1.18251418313119,-0.411552957311693,
1.23119764287622));
#49254=CARTESIAN_POINT('Ctrl Pts',(-1.23119764287622,-0.411552957311693,
1.18251418313119));
#49255=CARTESIAN_POINT('Ctrl Pts',(-1.25681160160691,-0.407041111792943,
1.15530234155453));
#49256=CARTESIAN_POINT('Ctrl Pts',(-1.30441816675528,-0.387888272594439,
1.10126842659597));
#49257=CARTESIAN_POINT('Ctrl Pts',(-1.32643091652006,-0.373243761060365,
1.07446535104584));
#49258=CARTESIAN_POINT('Ctrl Pts',(-1.36743459453896,-0.335108247315849,
1.02199477007745));
#49259=CARTESIAN_POINT('Ctrl Pts',(-1.39055359345152,-0.303141259068212,
0.990027513266106));
#49260=CARTESIAN_POINT('Ctrl Pts',(-1.4243271592157,-0.236152929235938,
0.940896403863071));
#49261=CARTESIAN_POINT('Ctrl Pts',(-1.43904931717599,-0.192480977588836,
0.917859913453974));
#49262=CARTESIAN_POINT('Ctrl Pts',(-1.45296717977858,-0.123823518623746,
0.895520212222106));
#49263=CARTESIAN_POINT('Ctrl Pts',(-1.45630208793976,-0.101649918886749,
0.890059788636852));
#49264=CARTESIAN_POINT('Ctrl Pts',(-1.45861320581289,-0.0793800000000001,
0.886256117232623));
#49265=CARTESIAN_POINT('',(-1.65807299932179,-0.07938,0.404717578595295));
#49266=CARTESIAN_POINT('Origin',(0.,-0.07938,0.));
#49267=CARTESIAN_POINT('',(-1.706752,-0.411552957311693,2.08591827245526E-16));
#49268=CARTESIAN_POINT('Ctrl Pts',(-1.65807299932179,-0.0793800000000001,
0.404717578595296));
#49269=CARTESIAN_POINT('Ctrl Pts',(-1.65912839404491,-0.101649918886749,
0.400393769631747));
#49270=CARTESIAN_POINT('Ctrl Pts',(-1.66063136041479,-0.123823518623745,
0.394174530911058));
#49271=CARTESIAN_POINT('Ctrl Pts',(-1.66658649961961,-0.192480977588835,
0.368536561654407));
#49272=CARTESIAN_POINT('Ctrl Pts',(-1.67246562047521,-0.236152929235937,
0.341837165343982));
#49273=CARTESIAN_POINT('Ctrl Pts',(-1.68332504372461,-0.303141259068211,
0.283214707341173));
#49274=CARTESIAN_POINT('Ctrl Pts',(-1.68958170688653,-0.335108247315848,
0.244262842368623));
#49275=CARTESIAN_POINT('Ctrl Pts',(-1.69769003172132,-0.373243761060364,
0.178166559972324));
#49276=CARTESIAN_POINT('Ctrl Pts',(-1.70107730356824,-0.387888272594439,
0.143648558862931));
#49277=CARTESIAN_POINT('Ctrl Pts',(-1.70562212620408,-0.407041111792943,
0.0717778861362656));
#49278=CARTESIAN_POINT('Ctrl Pts',(-1.706752,-0.411552957311693,0.0344244045173313));
#49279=CARTESIAN_POINT('Ctrl Pts',(-1.706752,-0.411552957311693,2.08166817117217E-16));
#49280=CARTESIAN_POINT('',(-1.706752,-0.47628,2.09016837373834E-16));
#49281=CARTESIAN_POINT('',(-1.706752,-0.27783,2.09016837373834E-16));
#49282=CARTESIAN_POINT('Origin',(0.,-0.47628,0.));
#49283=CARTESIAN_POINT('',(-1.65807299932179,-0.07938,-0.404717578595296));
#49284=CARTESIAN_POINT('Ctrl Pts',(-1.706752,-0.411552957311693,2.0122792321331E-16));
#49285=CARTESIAN_POINT('Ctrl Pts',(-1.706752,-0.411552957311693,-0.0344244045173309));
#49286=CARTESIAN_POINT('Ctrl Pts',(-1.70562212620408,-0.407041111792943,
-0.0717778861362652));
#49287=CARTESIAN_POINT('Ctrl Pts',(-1.70107730356824,-0.387888272594439,
-0.143648558862931));
#49288=CARTESIAN_POINT('Ctrl Pts',(-1.69769003172132,-0.373243761060365,
-0.178166559972324));
#49289=CARTESIAN_POINT('Ctrl Pts',(-1.68958170688653,-0.335108247315849,
-0.244262842368623));
#49290=CARTESIAN_POINT('Ctrl Pts',(-1.68332504372461,-0.303141259068212,
-0.283214707341173));
#49291=CARTESIAN_POINT('Ctrl Pts',(-1.67246562047521,-0.236152929235938,
-0.341837165343982));
#49292=CARTESIAN_POINT('Ctrl Pts',(-1.66658649961961,-0.192480977588836,
-0.368536561654407));
#49293=CARTESIAN_POINT('Ctrl Pts',(-1.66063136041479,-0.123823518623745,
-0.394174530911059));
#49294=CARTESIAN_POINT('Ctrl Pts',(-1.65912839404491,-0.101649918886749,
-0.400393769631748));
#49295=CARTESIAN_POINT('Ctrl Pts',(-1.65807299932179,-0.0793800000000001,
-0.404717578595296));
#49296=CARTESIAN_POINT('',(-1.45861320581289,-0.07938,-0.886256117232623));
#49297=CARTESIAN_POINT('Origin',(0.,-0.07938,0.));
#49298=CARTESIAN_POINT('',(-0.886256117232623,-0.07938,-1.45861320581289));
#49299=CARTESIAN_POINT('Ctrl Pts',(-1.45861320581289,-0.0793800000000001,
-0.886256117232623));
#49300=CARTESIAN_POINT('Ctrl Pts',(-1.45630208793976,-0.101649918886749,
-0.890059788636852));
#49301=CARTESIAN_POINT('Ctrl Pts',(-1.45296717977858,-0.123823518623745,
-0.895520212222106));
#49302=CARTESIAN_POINT('Ctrl Pts',(-1.43904931717599,-0.192480977588835,
-0.917859913453974));
#49303=CARTESIAN_POINT('Ctrl Pts',(-1.4243271592157,-0.236152929235937,
-0.940896403863072));
#49304=CARTESIAN_POINT('Ctrl Pts',(-1.39055359345152,-0.303141259068212,
-0.990027513266106));
#49305=CARTESIAN_POINT('Ctrl Pts',(-1.36743459453896,-0.335108247315849,
-1.02199477007745));
#49306=CARTESIAN_POINT('Ctrl Pts',(-1.32643091652006,-0.373243761060364,
-1.07446535104584));
#49307=CARTESIAN_POINT('Ctrl Pts',(-1.30441816675528,-0.387888272594439,
-1.10126842659597));
#49308=CARTESIAN_POINT('Ctrl Pts',(-1.25681160160691,-0.407041111792943,
-1.15530234155453));
#49309=CARTESIAN_POINT('Ctrl Pts',(-1.23119764287622,-0.411552957311693,
-1.18251418313119));
#49310=CARTESIAN_POINT('Ctrl Pts',(-1.18251418313119,-0.411552957311693,
-1.23119764287622));
#49311=CARTESIAN_POINT('Ctrl Pts',(-1.15530234155453,-0.407041111792943,
-1.25681160160691));
#49312=CARTESIAN_POINT('Ctrl Pts',(-1.10126842659597,-0.387888272594439,
-1.30441816675528));
#49313=CARTESIAN_POINT('Ctrl Pts',(-1.07446535104584,-0.373243761060364,
-1.32643091652006));
#49314=CARTESIAN_POINT('Ctrl Pts',(-1.02199477007745,-0.335108247315848,
-1.36743459453896));
#49315=CARTESIAN_POINT('Ctrl Pts',(-0.990027513266105,-0.303141259068211,
-1.39055359345152));
#49316=CARTESIAN_POINT('Ctrl Pts',(-0.940896403863071,-0.236152929235936,
-1.42432715921571));
#49317=CARTESIAN_POINT('Ctrl Pts',(-0.917859913453974,-0.192480977588835,
-1.43904931717599));
#49318=CARTESIAN_POINT('Ctrl Pts',(-0.895520212222106,-0.123823518623745,
-1.45296717977858));
#49319=CARTESIAN_POINT('Ctrl Pts',(-0.890059788636851,-0.101649918886749,
-1.45630208793976));
#49320=CARTESIAN_POINT('Ctrl Pts',(-0.886256117232623,-0.0793800000000001,
-1.45861320581289));
#49321=CARTESIAN_POINT('',(-0.404717578595295,-0.07938,-1.65807299932179));
#49322=CARTESIAN_POINT('Origin',(0.,-0.07938,0.));
#49323=CARTESIAN_POINT('',(0.404717578595296,-0.07938,-1.65807299932179));
#49324=CARTESIAN_POINT('Ctrl Pts',(-0.404717578595296,-0.0793800000000001,
-1.65807299932179));
#49325=CARTESIAN_POINT('Ctrl Pts',(-0.400393769631747,-0.101649918886749,
-1.65912839404491));
#49326=CARTESIAN_POINT('Ctrl Pts',(-0.394174530911058,-0.123823518623746,
-1.66063136041479));
#49327=CARTESIAN_POINT('Ctrl Pts',(-0.368536561654407,-0.192480977588836,
-1.66658649961961));
#49328=CARTESIAN_POINT('Ctrl Pts',(-0.341837165343982,-0.236152929235938,
-1.67246562047521));
#49329=CARTESIAN_POINT('Ctrl Pts',(-0.283214707341173,-0.303141259068212,
-1.68332504372461));
#49330=CARTESIAN_POINT('Ctrl Pts',(-0.244262842368623,-0.335108247315849,
-1.68958170688653));
#49331=CARTESIAN_POINT('Ctrl Pts',(-0.178166559972324,-0.373243761060364,
-1.69769003172132));
#49332=CARTESIAN_POINT('Ctrl Pts',(-0.143648558862931,-0.387888272594439,
-1.70107730356824));
#49333=CARTESIAN_POINT('Ctrl Pts',(-0.0717778861362653,-0.407041111792943,
-1.70562212620408));
#49334=CARTESIAN_POINT('Ctrl Pts',(-0.034424404517331,-0.411552957311693,
-1.706752));
#49335=CARTESIAN_POINT('Ctrl Pts',(0.0344244045173312,-0.411552957311693,
-1.706752));
#49336=CARTESIAN_POINT('Ctrl Pts',(0.0717778861362655,-0.407041111792943,
-1.70562212620408));
#49337=CARTESIAN_POINT('Ctrl Pts',(0.143648558862931,-0.387888272594439,
-1.70107730356824));
#49338=CARTESIAN_POINT('Ctrl Pts',(0.178166559972324,-0.373243761060364,
-1.69769003172132));
#49339=CARTESIAN_POINT('Ctrl Pts',(0.244262842368623,-0.335108247315849,
-1.68958170688653));
#49340=CARTESIAN_POINT('Ctrl Pts',(0.283214707341173,-0.303141259068212,
-1.68332504372461));
#49341=CARTESIAN_POINT('Ctrl Pts',(0.341837165343982,-0.236152929235937,
-1.67246562047521));
#49342=CARTESIAN_POINT('Ctrl Pts',(0.368536561654407,-0.192480977588835,
-1.66658649961961));
#49343=CARTESIAN_POINT('Ctrl Pts',(0.394174530911059,-0.123823518623745,
-1.66063136041479));
#49344=CARTESIAN_POINT('Ctrl Pts',(0.400393769631748,-0.101649918886749,
-1.65912839404491));
#49345=CARTESIAN_POINT('Ctrl Pts',(0.404717578595296,-0.0793800000000001,
-1.65807299932179));
#49346=CARTESIAN_POINT('',(0.886256117232623,-0.07938,-1.45861320581289));
#49347=CARTESIAN_POINT('Origin',(0.,-0.07938,0.));
#49348=CARTESIAN_POINT('',(1.45861320581289,-0.07938,-0.886256117232623));
#49349=CARTESIAN_POINT('Ctrl Pts',(0.886256117232623,-0.0793800000000001,
-1.45861320581289));
#49350=CARTESIAN_POINT('Ctrl Pts',(0.890059788636852,-0.101649918886749,
-1.45630208793976));
#49351=CARTESIAN_POINT('Ctrl Pts',(0.895520212222106,-0.123823518623745,
-1.45296717977858));
#49352=CARTESIAN_POINT('Ctrl Pts',(0.917859913453974,-0.192480977588835,
-1.43904931717599));
#49353=CARTESIAN_POINT('Ctrl Pts',(0.940896403863072,-0.236152929235937,
-1.4243271592157));
#49354=CARTESIAN_POINT('Ctrl Pts',(0.990027513266106,-0.303141259068211,
-1.39055359345152));
#49355=CARTESIAN_POINT('Ctrl Pts',(1.02199477007745,-0.335108247315849,
-1.36743459453896));
#49356=CARTESIAN_POINT('Ctrl Pts',(1.07446535104584,-0.373243761060364,
-1.32643091652006));
#49357=CARTESIAN_POINT('Ctrl Pts',(1.10126842659597,-0.387888272594439,
-1.30441816675528));
#49358=CARTESIAN_POINT('Ctrl Pts',(1.15530234155453,-0.407041111792943,
-1.25681160160691));
#49359=CARTESIAN_POINT('Ctrl Pts',(1.18251418313119,-0.411552957311693,
-1.23119764287622));
#49360=CARTESIAN_POINT('Ctrl Pts',(1.23119764287622,-0.411552957311693,
-1.18251418313119));
#49361=CARTESIAN_POINT('Ctrl Pts',(1.25681160160691,-0.407041111792943,
-1.15530234155453));
#49362=CARTESIAN_POINT('Ctrl Pts',(1.30441816675528,-0.387888272594439,
-1.10126842659597));
#49363=CARTESIAN_POINT('Ctrl Pts',(1.32643091652006,-0.373243761060364,
-1.07446535104584));
#49364=CARTESIAN_POINT('Ctrl Pts',(1.36743459453896,-0.335108247315849,
-1.02199477007745));
#49365=CARTESIAN_POINT('Ctrl Pts',(1.39055359345152,-0.303141259068212,
-0.990027513266105));
#49366=CARTESIAN_POINT('Ctrl Pts',(1.4243271592157,-0.236152929235937,-0.940896403863071));
#49367=CARTESIAN_POINT('Ctrl Pts',(1.43904931717599,-0.192480977588835,
-0.917859913453974));
#49368=CARTESIAN_POINT('Ctrl Pts',(1.45296717977858,-0.123823518623745,
-0.895520212222106));
#49369=CARTESIAN_POINT('Ctrl Pts',(1.45630208793976,-0.101649918886749,
-0.890059788636852));
#49370=CARTESIAN_POINT('Ctrl Pts',(1.45861320581289,-0.0793800000000001,
-0.886256117232623));
#49371=CARTESIAN_POINT('',(1.65807299932179,-0.07938,-0.404717578595296));
#49372=CARTESIAN_POINT('Origin',(0.,-0.07938,0.));
#49373=CARTESIAN_POINT('',(1.65807299932179,-0.07938,0.404717578595296));
#49374=CARTESIAN_POINT('Ctrl Pts',(1.65807299932179,-0.0793800000000001,
-0.404717578595296));
#49375=CARTESIAN_POINT('Ctrl Pts',(1.65912839404491,-0.101649918886749,
-0.400393769631747));
#49376=CARTESIAN_POINT('Ctrl Pts',(1.66063136041479,-0.123823518623745,
-0.394174530911058));
#49377=CARTESIAN_POINT('Ctrl Pts',(1.66658649961961,-0.192480977588835,
-0.368536561654407));
#49378=CARTESIAN_POINT('Ctrl Pts',(1.67246562047521,-0.236152929235937,
-0.341837165343982));
#49379=CARTESIAN_POINT('Ctrl Pts',(1.68332504372461,-0.303141259068212,
-0.283214707341173));
#49380=CARTESIAN_POINT('Ctrl Pts',(1.68958170688653,-0.335108247315849,
-0.244262842368623));
#49381=CARTESIAN_POINT('Ctrl Pts',(1.69769003172132,-0.373243761060364,
-0.178166559972324));
#49382=CARTESIAN_POINT('Ctrl Pts',(1.70107730356824,-0.387888272594439,
-0.143648558862931));
#49383=CARTESIAN_POINT('Ctrl Pts',(1.70562212620408,-0.407041111792943,
-0.0717778861362655));
#49384=CARTESIAN_POINT('Ctrl Pts',(1.706752,-0.411552957311693,-0.0344244045173312));
#49385=CARTESIAN_POINT('Ctrl Pts',(1.706752,-0.411552957311693,0.0344244045173312));
#49386=CARTESIAN_POINT('Ctrl Pts',(1.70562212620408,-0.407041111792943,
0.0717778861362655));
#49387=CARTESIAN_POINT('Ctrl Pts',(1.70107730356824,-0.387888272594439,
0.143648558862931));
#49388=CARTESIAN_POINT('Ctrl Pts',(1.69769003172132,-0.373243761060364,
0.178166559972324));
#49389=CARTESIAN_POINT('Ctrl Pts',(1.68958170688653,-0.335108247315849,
0.244262842368623));
#49390=CARTESIAN_POINT('Ctrl Pts',(1.68332504372461,-0.303141259068212,
0.283214707341173));
#49391=CARTESIAN_POINT('Ctrl Pts',(1.67246562047521,-0.236152929235937,
0.341837165343982));
#49392=CARTESIAN_POINT('Ctrl Pts',(1.66658649961961,-0.192480977588835,
0.368536561654407));
#49393=CARTESIAN_POINT('Ctrl Pts',(1.66063136041479,-0.123823518623745,
0.394174530911058));
#49394=CARTESIAN_POINT('Ctrl Pts',(1.65912839404491,-0.101649918886749,
0.400393769631747));
#49395=CARTESIAN_POINT('Ctrl Pts',(1.65807299932179,-0.0793800000000001,
0.404717578595296));
#49396=CARTESIAN_POINT('Origin',(0.,-0.07938,0.));
#49397=CARTESIAN_POINT('Origin',(0.,-0.07938,0.));
#49398=CARTESIAN_POINT('',(0.397005914195118,-0.07938,1.59456899932179));
#49399=CARTESIAN_POINT('Origin',(0.,-0.07938,0.));
#49400=CARTESIAN_POINT('Origin',(-3.33066907387547E-16,-0.07938,1.675));
#49401=CARTESIAN_POINT('Origin',(-3.33066907387547E-16,0.,1.675));
#49402=CARTESIAN_POINT('',(-0.397005914195118,-0.07938,1.59456899932179));
#49403=CARTESIAN_POINT('Ctrl Pts',(-0.397005914195119,-0.0793800000000001,
1.59456899932179));
#49404=CARTESIAN_POINT('Ctrl Pts',(-0.3886265584581,-0.123401821157026,
1.59665523941937));
#49405=CARTESIAN_POINT('Ctrl Pts',(-0.373030350867485,-0.166543350814306,
1.60050712143809));
#49406=CARTESIAN_POINT('Ctrl Pts',(-0.333298652394954,-0.237231147975234,
1.60919314384089));
#49407=CARTESIAN_POINT('Ctrl Pts',(-0.311480544243687,-0.266264900654909,
1.61365775139403));
#49408=CARTESIAN_POINT('Ctrl Pts',(-0.261368388670537,-0.317195968905306,
1.62252828437015));
#49409=CARTESIAN_POINT('Ctrl Pts',(-0.233069203882014,-0.33909093068465,
1.62691869420078));
#49410=CARTESIAN_POINT('Ctrl Pts',(-0.174042761838764,-0.373586846396559,
1.63426473152765));
#49411=CARTESIAN_POINT('Ctrl Pts',(-0.14036578147155,-0.388086240756494,
1.63761964365402));
#49412=CARTESIAN_POINT('Ctrl Pts',(-0.0701778381840615,-0.407068917407805,
1.64212536811722));
#49413=CARTESIAN_POINT('Ctrl Pts',(-0.0336652739555918,-0.411552957311693,
1.643248));
#49414=CARTESIAN_POINT('Ctrl Pts',(0.0336652739555913,-0.411552957311693,
1.643248));
#49415=CARTESIAN_POINT('Ctrl Pts',(0.070177838184061,-0.407068917407805,
1.64212536811722));
#49416=CARTESIAN_POINT('Ctrl Pts',(0.140365781471549,-0.388086240756494,
1.63761964365402));
#49417=CARTESIAN_POINT('Ctrl Pts',(0.174042761838763,-0.373586846396559,
1.63426473152765));
#49418=CARTESIAN_POINT('Ctrl Pts',(0.233069203882014,-0.33909093068465,
1.62691869420078));
#49419=CARTESIAN_POINT('Ctrl Pts',(0.261368388670536,-0.317195968905306,
1.62252828437015));
#49420=CARTESIAN_POINT('Ctrl Pts',(0.311480544243686,-0.266264900654908,
1.61365775139403));
#49421=CARTESIAN_POINT('Ctrl Pts',(0.333298652394954,-0.237231147975234,
1.60919314384089));
#49422=CARTESIAN_POINT('Ctrl Pts',(0.373030350867484,-0.166543350814306,
1.60050712143809));
#49423=CARTESIAN_POINT('Ctrl Pts',(0.388626558458099,-0.123401821157026,
1.59665523941937));
#49424=CARTESIAN_POINT('Ctrl Pts',(0.397005914195118,-0.07938,1.59456899932179));
#49425=CARTESIAN_POINT('Origin',(-3.33066907387547E-16,-0.07938,1.675));
#49426=CARTESIAN_POINT('Origin',(0.,-0.07938,0.));
#49427=CARTESIAN_POINT('',(-0.846804978391754,-0.07938,1.40825612658882));
#49428=CARTESIAN_POINT('Origin',(0.,-0.07938,0.));
#49429=CARTESIAN_POINT('Origin',(-1.18440385848747,-0.07938,1.18440385848747));
#49430=CARTESIAN_POINT('Origin',(-1.18440385848747,0.,1.18440385848747));
#49431=CARTESIAN_POINT('',(-1.40825612658882,-0.07938,0.846804978391753));
#49432=CARTESIAN_POINT('Ctrl Pts',(-1.40825612658882,-0.0793800000000001,
0.846804978391753));
#49433=CARTESIAN_POINT('Ctrl Pts',(-1.40380622184538,-0.123401821157026,
0.854205272175555));
#49434=CARTESIAN_POINT('Ctrl Pts',(-1.39550172959303,-0.166543350814306,
0.867957148219442));
#49435=CARTESIAN_POINT('Ctrl Pts',(-1.3735491215176,-0.237231147975235,
0.902193646979983));
#49436=CARTESIAN_POINT('Ctrl Pts',(-1.36127834356734,-0.266264900654909,
0.920778333482565));
#49437=CARTESIAN_POINT('Ctrl Pts',(-1.33211611256184,-0.317195968905306,
0.962485392528369));
#49438=CARTESIAN_POINT('Ctrl Pts',(-1.31521005565926,-0.339090930684651,
0.985600426557816));
#49439=CARTESIAN_POINT('Ctrl Pts',(-1.27866649102984,-0.373586846396559,
1.03253285680459));
#49440=CARTESIAN_POINT('Ctrl Pts',(-1.25722555095714,-0.388086240756494,
1.05871835910697));
#49441=CARTESIAN_POINT('Ctrl Pts',(-1.2107812086231,-0.407068917407805,
1.11153475808518));
#49442=CARTESIAN_POINT('Ctrl Pts',(-1.18575674747573,-0.411552957311693,
1.13814686046673));
#49443=CARTESIAN_POINT('Ctrl Pts',(-1.13814686046673,-0.411552957311693,
1.18575674747573));
#49444=CARTESIAN_POINT('Ctrl Pts',(-1.11153475808518,-0.407068917407805,
1.2107812086231));
#49445=CARTESIAN_POINT('Ctrl Pts',(-1.05871835910697,-0.388086240756494,
1.25722555095714));
#49446=CARTESIAN_POINT('Ctrl Pts',(-1.03253285680459,-0.373586846396559,
1.27866649102984));
#49447=CARTESIAN_POINT('Ctrl Pts',(-0.985600426557816,-0.33909093068465,
1.31521005565926));
#49448=CARTESIAN_POINT('Ctrl Pts',(-0.962485392528369,-0.317195968905306,
1.33211611256184));
#49449=CARTESIAN_POINT('Ctrl Pts',(-0.920778333482565,-0.266264900654908,
1.36127834356734));
#49450=CARTESIAN_POINT('Ctrl Pts',(-0.902193646979983,-0.237231147975234,
1.3735491215176));
#49451=CARTESIAN_POINT('Ctrl Pts',(-0.867957148219442,-0.166543350814306,
1.39550172959303));
#49452=CARTESIAN_POINT('Ctrl Pts',(-0.854205272175555,-0.123401821157026,
1.40380622184538));
#49453=CARTESIAN_POINT('Ctrl Pts',(-0.846804978391753,-0.0793800000000001,
1.40825612658882));
#49454=CARTESIAN_POINT('Origin',(-1.18440385848747,-0.07938,1.18440385848747));
#49455=CARTESIAN_POINT('Origin',(0.,-0.07938,0.));
#49456=CARTESIAN_POINT('',(-1.59456899932179,-0.07938,0.397005914195118));
#49457=CARTESIAN_POINT('Origin',(0.,-0.07938,0.));
#49458=CARTESIAN_POINT('Origin',(-1.675,-0.07938,-2.22044604925031E-16));
#49459=CARTESIAN_POINT('Origin',(-1.675,0.,-2.22044604925031E-16));
#49460=CARTESIAN_POINT('',(-1.59456899932179,-0.07938,-0.397005914195118));
#49461=CARTESIAN_POINT('',(-1.643248,-0.411552957311693,3.47540551556327E-18));
#49462=CARTESIAN_POINT('Ctrl Pts',(-1.59456899932179,-0.0793800000000001,
-0.397005914195119));
#49463=CARTESIAN_POINT('Ctrl Pts',(-1.59665523941937,-0.123401821157026,
-0.388626558458099));
#49464=CARTESIAN_POINT('Ctrl Pts',(-1.60050712143809,-0.166543350814306,
-0.373030350867485));
#49465=CARTESIAN_POINT('Ctrl Pts',(-1.60919314384089,-0.237231147975234,
-0.333298652394954));
#49466=CARTESIAN_POINT('Ctrl Pts',(-1.61365775139403,-0.266264900654909,
-0.311480544243686));
#49467=CARTESIAN_POINT('Ctrl Pts',(-1.62252828437015,-0.317195968905306,
-0.261368388670537));
#49468=CARTESIAN_POINT('Ctrl Pts',(-1.62691869420078,-0.33909093068465,
-0.233069203882014));
#49469=CARTESIAN_POINT('Ctrl Pts',(-1.63426473152765,-0.373586846396559,
-0.174042761838764));
#49470=CARTESIAN_POINT('Ctrl Pts',(-1.63761964365402,-0.388086240756494,
-0.140365781471549));
#49471=CARTESIAN_POINT('Ctrl Pts',(-1.64212536811722,-0.407068917407805,
-0.0701778381840614));
#49472=CARTESIAN_POINT('Ctrl Pts',(-1.643248,-0.411552957311693,-0.0336652739555917));
#49473=CARTESIAN_POINT('Ctrl Pts',(-1.643248,-0.411552957311693,-2.0122792321331E-16));
#49474=CARTESIAN_POINT('Origin',(-1.675,-0.07938,-2.22044604925031E-16));
#49475=CARTESIAN_POINT('Ctrl Pts',(-1.643248,-0.411552957311693,-1.94289029309402E-16));
#49476=CARTESIAN_POINT('Ctrl Pts',(-1.643248,-0.411552957311693,0.0336652739555913));
#49477=CARTESIAN_POINT('Ctrl Pts',(-1.64212536811722,-0.407068917407805,
0.0701778381840609));
#49478=CARTESIAN_POINT('Ctrl Pts',(-1.63761964365402,-0.388086240756494,
0.140365781471549));
#49479=CARTESIAN_POINT('Ctrl Pts',(-1.63426473152765,-0.373586846396559,
0.174042761838763));
#49480=CARTESIAN_POINT('Ctrl Pts',(-1.62691869420078,-0.33909093068465,
0.233069203882014));
#49481=CARTESIAN_POINT('Ctrl Pts',(-1.62252828437015,-0.317195968905306,
0.261368388670536));
#49482=CARTESIAN_POINT('Ctrl Pts',(-1.61365775139403,-0.266264900654909,
0.311480544243686));
#49483=CARTESIAN_POINT('Ctrl Pts',(-1.60919314384089,-0.237231147975235,
0.333298652394954));
#49484=CARTESIAN_POINT('Ctrl Pts',(-1.60050712143809,-0.166543350814306,
0.373030350867484));
#49485=CARTESIAN_POINT('Ctrl Pts',(-1.59665523941937,-0.123401821157026,
0.388626558458099));
#49486=CARTESIAN_POINT('Ctrl Pts',(-1.59456899932179,-0.0793800000000001,
0.397005914195118));
#49487=CARTESIAN_POINT('Origin',(0.,-0.07938,0.));
#49488=CARTESIAN_POINT('',(-1.40825612658882,-0.07938,-0.846804978391753));
#49489=CARTESIAN_POINT('Origin',(0.,-0.07938,0.));
#49490=CARTESIAN_POINT('Origin',(-1.18440385848747,-0.07938,-1.18440385848747));
#49491=CARTESIAN_POINT('Origin',(-1.18440385848747,0.,-1.18440385848747));
#49492=CARTESIAN_POINT('',(-0.846804978391753,-0.07938,-1.40825612658882));
#49493=CARTESIAN_POINT('Ctrl Pts',(-0.846804978391753,-0.0793800000000001,
-1.40825612658882));
#49494=CARTESIAN_POINT('Ctrl Pts',(-0.854205272175555,-0.123401821157026,
-1.40380622184538));
#49495=CARTESIAN_POINT('Ctrl Pts',(-0.867957148219442,-0.166543350814306,
-1.39550172959303));
#49496=CARTESIAN_POINT('Ctrl Pts',(-0.902193646979982,-0.237231147975234,
-1.3735491215176));
#49497=CARTESIAN_POINT('Ctrl Pts',(-0.920778333482564,-0.266264900654908,
-1.36127834356734));
#49498=CARTESIAN_POINT('Ctrl Pts',(-0.962485392528368,-0.317195968905306,
-1.33211611256184));
#49499=CARTESIAN_POINT('Ctrl Pts',(-0.985600426557816,-0.33909093068465,
-1.31521005565926));
#49500=CARTESIAN_POINT('Ctrl Pts',(-1.03253285680459,-0.373586846396559,
-1.27866649102984));
#49501=CARTESIAN_POINT('Ctrl Pts',(-1.05871835910697,-0.388086240756494,
-1.25722555095714));
#49502=CARTESIAN_POINT('Ctrl Pts',(-1.11153475808518,-0.407068917407805,
-1.2107812086231));
#49503=CARTESIAN_POINT('Ctrl Pts',(-1.13814686046673,-0.411552957311693,
-1.18575674747573));
#49504=CARTESIAN_POINT('Ctrl Pts',(-1.18575674747573,-0.411552957311693,
-1.13814686046673));
#49505=CARTESIAN_POINT('Ctrl Pts',(-1.2107812086231,-0.407068917407805,
-1.11153475808518));
#49506=CARTESIAN_POINT('Ctrl Pts',(-1.25722555095714,-0.388086240756494,
-1.05871835910697));
#49507=CARTESIAN_POINT('Ctrl Pts',(-1.27866649102984,-0.373586846396559,
-1.03253285680459));
#49508=CARTESIAN_POINT('Ctrl Pts',(-1.31521005565926,-0.33909093068465,
-0.985600426557816));
#49509=CARTESIAN_POINT('Ctrl Pts',(-1.33211611256184,-0.317195968905306,
-0.962485392528369));
#49510=CARTESIAN_POINT('Ctrl Pts',(-1.36127834356734,-0.266264900654909,
-0.920778333482565));
#49511=CARTESIAN_POINT('Ctrl Pts',(-1.3735491215176,-0.237231147975234,
-0.902193646979983));
#49512=CARTESIAN_POINT('Ctrl Pts',(-1.39550172959303,-0.166543350814306,
-0.867957148219442));
#49513=CARTESIAN_POINT('Ctrl Pts',(-1.40380622184538,-0.123401821157026,
-0.854205272175555));
#49514=CARTESIAN_POINT('Ctrl Pts',(-1.40825612658882,-0.07938,-0.846804978391753));
#49515=CARTESIAN_POINT('Origin',(-1.18440385848747,-0.07938,-1.18440385848747));
#49516=CARTESIAN_POINT('Origin',(0.,-0.07938,0.));
#49517=CARTESIAN_POINT('',(-0.397005914195118,-0.07938,-1.59456899932179));
#49518=CARTESIAN_POINT('Origin',(0.,-0.07938,0.));
#49519=CARTESIAN_POINT('Origin',(1.11022302462516E-16,-0.07938,-1.675));
#49520=CARTESIAN_POINT('Origin',(1.11022302462516E-16,0.,-1.675));
#49521=CARTESIAN_POINT('',(0.397005914195118,-0.07938,-1.59456899932179));
#49522=CARTESIAN_POINT('Ctrl Pts',(0.397005914195119,-0.0793800000000001,
-1.59456899932179));
#49523=CARTESIAN_POINT('Ctrl Pts',(0.388626558458099,-0.123401821157026,
-1.59665523941937));
#49524=CARTESIAN_POINT('Ctrl Pts',(0.373030350867485,-0.166543350814306,
-1.60050712143809));
#49525=CARTESIAN_POINT('Ctrl Pts',(0.333298652394954,-0.237231147975234,
-1.60919314384089));
#49526=CARTESIAN_POINT('Ctrl Pts',(0.311480544243686,-0.266264900654909,
-1.61365775139403));
#49527=CARTESIAN_POINT('Ctrl Pts',(0.261368388670537,-0.317195968905306,
-1.62252828437015));
#49528=CARTESIAN_POINT('Ctrl Pts',(0.233069203882014,-0.33909093068465,
-1.62691869420078));
#49529=CARTESIAN_POINT('Ctrl Pts',(0.174042761838763,-0.373586846396559,
-1.63426473152765));
#49530=CARTESIAN_POINT('Ctrl Pts',(0.140365781471549,-0.388086240756494,
-1.63761964365402));
#49531=CARTESIAN_POINT('Ctrl Pts',(0.0701778381840612,-0.407068917407805,
-1.64212536811722));
#49532=CARTESIAN_POINT('Ctrl Pts',(0.0336652739555916,-0.411552957311693,
-1.643248));
#49533=CARTESIAN_POINT('Ctrl Pts',(-0.0336652739555915,-0.411552957311693,
-1.643248));
#49534=CARTESIAN_POINT('Ctrl Pts',(-0.0701778381840612,-0.407068917407805,
-1.64212536811722));
#49535=CARTESIAN_POINT('Ctrl Pts',(-0.140365781471549,-0.388086240756494,
-1.63761964365402));
#49536=CARTESIAN_POINT('Ctrl Pts',(-0.174042761838764,-0.373586846396559,
-1.63426473152765));
#49537=CARTESIAN_POINT('Ctrl Pts',(-0.233069203882014,-0.33909093068465,
-1.62691869420078));
#49538=CARTESIAN_POINT('Ctrl Pts',(-0.261368388670536,-0.317195968905306,
-1.62252828437015));
#49539=CARTESIAN_POINT('Ctrl Pts',(-0.311480544243686,-0.266264900654908,
-1.61365775139403));
#49540=CARTESIAN_POINT('Ctrl Pts',(-0.333298652394954,-0.237231147975234,
-1.60919314384089));
#49541=CARTESIAN_POINT('Ctrl Pts',(-0.373030350867485,-0.166543350814306,
-1.60050712143809));
#49542=CARTESIAN_POINT('Ctrl Pts',(-0.388626558458099,-0.123401821157026,
-1.59665523941937));
#49543=CARTESIAN_POINT('Ctrl Pts',(-0.397005914195118,-0.07938,-1.59456899932179));
#49544=CARTESIAN_POINT('Origin',(1.11022302462516E-16,-0.07938,-1.675));
#49545=CARTESIAN_POINT('Origin',(0.,-0.07938,0.));
#49546=CARTESIAN_POINT('',(0.846804978391753,-0.07938,-1.40825612658882));
#49547=CARTESIAN_POINT('Origin',(0.,-0.07938,0.));
#49548=CARTESIAN_POINT('Origin',(1.18440385848747,-0.07938,-1.18440385848747));
#49549=CARTESIAN_POINT('Origin',(1.18440385848747,0.,-1.18440385848747));
#49550=CARTESIAN_POINT('',(1.40825612658882,-0.07938,-0.846804978391753));
#49551=CARTESIAN_POINT('Ctrl Pts',(1.40825612658882,-0.0793800000000001,
-0.846804978391753));
#49552=CARTESIAN_POINT('Ctrl Pts',(1.40380622184538,-0.123401821157026,
-0.854205272175555));
#49553=CARTESIAN_POINT('Ctrl Pts',(1.39550172959303,-0.166543350814306,
-0.867957148219442));
#49554=CARTESIAN_POINT('Ctrl Pts',(1.3735491215176,-0.237231147975234,-0.902193646979983));
#49555=CARTESIAN_POINT('Ctrl Pts',(1.36127834356734,-0.266264900654908,
-0.920778333482565));
#49556=CARTESIAN_POINT('Ctrl Pts',(1.33211611256184,-0.317195968905306,
-0.962485392528369));
#49557=CARTESIAN_POINT('Ctrl Pts',(1.31521005565926,-0.33909093068465,-0.985600426557816));
#49558=CARTESIAN_POINT('Ctrl Pts',(1.27866649102984,-0.373586846396559,
-1.03253285680459));
#49559=CARTESIAN_POINT('Ctrl Pts',(1.25722555095714,-0.388086240756494,
-1.05871835910697));
#49560=CARTESIAN_POINT('Ctrl Pts',(1.2107812086231,-0.407068917407805,-1.11153475808518));
#49561=CARTESIAN_POINT('Ctrl Pts',(1.18575674747573,-0.411552957311693,
-1.13814686046673));
#49562=CARTESIAN_POINT('Ctrl Pts',(1.13814686046673,-0.411552957311693,
-1.18575674747573));
#49563=CARTESIAN_POINT('Ctrl Pts',(1.11153475808518,-0.407068917407805,
-1.2107812086231));
#49564=CARTESIAN_POINT('Ctrl Pts',(1.05871835910697,-0.388086240756494,
-1.25722555095714));
#49565=CARTESIAN_POINT('Ctrl Pts',(1.03253285680459,-0.373586846396559,
-1.27866649102984));
#49566=CARTESIAN_POINT('Ctrl Pts',(0.985600426557816,-0.33909093068465,
-1.31521005565926));
#49567=CARTESIAN_POINT('Ctrl Pts',(0.962485392528369,-0.317195968905306,
-1.33211611256184));
#49568=CARTESIAN_POINT('Ctrl Pts',(0.920778333482565,-0.266264900654909,
-1.36127834356734));
#49569=CARTESIAN_POINT('Ctrl Pts',(0.902193646979983,-0.237231147975234,
-1.3735491215176));
#49570=CARTESIAN_POINT('Ctrl Pts',(0.867957148219442,-0.166543350814306,
-1.39550172959303));
#49571=CARTESIAN_POINT('Ctrl Pts',(0.854205272175555,-0.123401821157026,
-1.40380622184538));
#49572=CARTESIAN_POINT('Ctrl Pts',(0.846804978391753,-0.0793800000000001,
-1.40825612658882));
#49573=CARTESIAN_POINT('Origin',(1.18440385848747,-0.07938,-1.18440385848747));
#49574=CARTESIAN_POINT('Origin',(0.,-0.27783,0.));
#49575=CARTESIAN_POINT('',(-1.643248,-0.47628,2.01239840340529E-16));
#49576=CARTESIAN_POINT('Origin',(0.,-0.47628,0.));
#49577=CARTESIAN_POINT('',(-1.643248,-0.27783,2.01239840340529E-16));
#49578=CARTESIAN_POINT('',(1.59456899932179,-0.07938,0.397005914195118));
#49579=CARTESIAN_POINT('Origin',(0.,-0.07938,0.));
#49580=CARTESIAN_POINT('',(1.59456899932179,-0.07938,-0.397005914195118));
#49581=CARTESIAN_POINT('Ctrl Pts',(1.59456899932179,-0.0793800000000001,
0.397005914195118));
#49582=CARTESIAN_POINT('Ctrl Pts',(1.59665523941937,-0.123401821157026,
0.388626558458099));
#49583=CARTESIAN_POINT('Ctrl Pts',(1.60050712143809,-0.166543350814306,
0.373030350867485));
#49584=CARTESIAN_POINT('Ctrl Pts',(1.60919314384089,-0.237231147975234,
0.333298652394954));
#49585=CARTESIAN_POINT('Ctrl Pts',(1.61365775139403,-0.266264900654909,
0.311480544243686));
#49586=CARTESIAN_POINT('Ctrl Pts',(1.62252828437015,-0.317195968905306,
0.261368388670537));
#49587=CARTESIAN_POINT('Ctrl Pts',(1.62691869420078,-0.33909093068465,0.233069203882014));
#49588=CARTESIAN_POINT('Ctrl Pts',(1.63426473152765,-0.373586846396559,
0.174042761838764));
#49589=CARTESIAN_POINT('Ctrl Pts',(1.63761964365402,-0.388086240756494,
0.140365781471549));
#49590=CARTESIAN_POINT('Ctrl Pts',(1.64212536811722,-0.407068917407805,
0.0701778381840612));
#49591=CARTESIAN_POINT('Ctrl Pts',(1.643248,-0.411552957311693,0.0336652739555916));
#49592=CARTESIAN_POINT('Ctrl Pts',(1.643248,-0.411552957311693,-0.0336652739555916));
#49593=CARTESIAN_POINT('Ctrl Pts',(1.64212536811722,-0.407068917407805,
-0.0701778381840612));
#49594=CARTESIAN_POINT('Ctrl Pts',(1.63761964365402,-0.388086240756494,
-0.140365781471549));
#49595=CARTESIAN_POINT('Ctrl Pts',(1.63426473152765,-0.373586846396559,
-0.174042761838764));
#49596=CARTESIAN_POINT('Ctrl Pts',(1.62691869420078,-0.33909093068465,-0.233069203882014));
#49597=CARTESIAN_POINT('Ctrl Pts',(1.62252828437015,-0.317195968905306,
-0.261368388670537));
#49598=CARTESIAN_POINT('Ctrl Pts',(1.61365775139403,-0.266264900654909,
-0.311480544243686));
#49599=CARTESIAN_POINT('Ctrl Pts',(1.60919314384089,-0.237231147975234,
-0.333298652394954));
#49600=CARTESIAN_POINT('Ctrl Pts',(1.60050712143809,-0.166543350814306,
-0.373030350867485));
#49601=CARTESIAN_POINT('Ctrl Pts',(1.59665523941937,-0.123401821157026,
-0.388626558458099));
#49602=CARTESIAN_POINT('Ctrl Pts',(1.59456899932179,-0.07938,-0.397005914195118));
#49603=CARTESIAN_POINT('Origin',(0.,-0.07938,0.));
#49604=CARTESIAN_POINT('Origin',(0.,-0.07938,0.));
#49605=CARTESIAN_POINT('Origin',(1.675,-0.07938,0.));
#49606=CARTESIAN_POINT('Origin',(1.675,0.,0.));
#49607=CARTESIAN_POINT('Origin',(1.675,-0.07938,0.));
#49608=CARTESIAN_POINT('Origin',(0.,-0.47628,0.));
#49609=CARTESIAN_POINT('Origin',(0.,-0.07938,0.));
#62858=UNCERTAINTY_MEASURE_WITH_UNIT(LENGTH_MEASURE(0.001),#62985,
'DISTANCE_ACCURACY_VALUE',
'Maximum model space distance between geometric entities at asserted c
onnectivities');
#62885=UNCERTAINTY_MEASURE_WITH_UNIT(LENGTH_MEASURE(0.001),#62985,
'DISTANCE_ACCURACY_VALUE',
'Maximum model space distance between geometric entities at asserted c
onnectivities');
#62957=(
GEOMETRIC_REPRESENTATION_CONTEXT(3)
GLOBAL_UNCERTAINTY_ASSIGNED_CONTEXT((#62858))
GLOBAL_UNIT_ASSIGNED_CONTEXT((#62985,#62987,#62988))
REPRESENTATION_CONTEXT('','3D')
);
#62984=(
GEOMETRIC_REPRESENTATION_CONTEXT(3)
GLOBAL_UNCERTAINTY_ASSIGNED_CONTEXT((#62885))
GLOBAL_UNIT_ASSIGNED_CONTEXT((#62985,#62987,#62988))
REPRESENTATION_CONTEXT('','3D')
);
#62985=(
LENGTH_UNIT()
NAMED_UNIT(*)
SI_UNIT(.CENTI.,.METRE.)
);
#62987=(
NAMED_UNIT(*)
PLANE_ANGLE_UNIT()
SI_UNIT($,.RADIAN.)
);
#62988=(
NAMED_UNIT(*)
SI_UNIT($,.STERADIAN.)
SOLID_ANGLE_UNIT()
);
#63060=SHAPE_DEFINITION_REPRESENTATION(#63243,#63420);
#63243=PRODUCT_DEFINITION_SHAPE('',$,#63519);
#63420=SHAPE_REPRESENTATION('',(#25716),#62957);
#63447=PRODUCT_DEFINITION_CONTEXT('part definition',#63743,'design');
#63519=PRODUCT_DEFINITION('Cage (1) (1)','Cage (1) (1)',#63617,#63447);
#63617=PRODUCT_DEFINITION_FORMATION('',$,#63816);
#63743=APPLICATION_CONTEXT(
'Core Data for Automotive Mechanical Design Process');
#63744=PRODUCT_CONTEXT('part definition',#63743,'mechanical');
#63816=PRODUCT('Cage (1) (1)','Cage (1) (1)','Cage (1) (1)',(#63744));
#63920=COLOUR_RGB('Off White',0.89,0.88,0.83);
#63921=FILL_AREA_STYLE_COLOUR('',#63920);
#63922=FILL_AREA_STYLE('',(#63921));
#63923=SURFACE_STYLE_FILL_AREA(#63922);
#63924=SURFACE_SIDE_STYLE('',(#63923));
#63925=SURFACE_STYLE_USAGE(.BOTH.,#63924);
#63926=PRESENTATION_STYLE_ASSIGNMENT((#63925));
ENDSEC;
END-ISO-10303-21;
